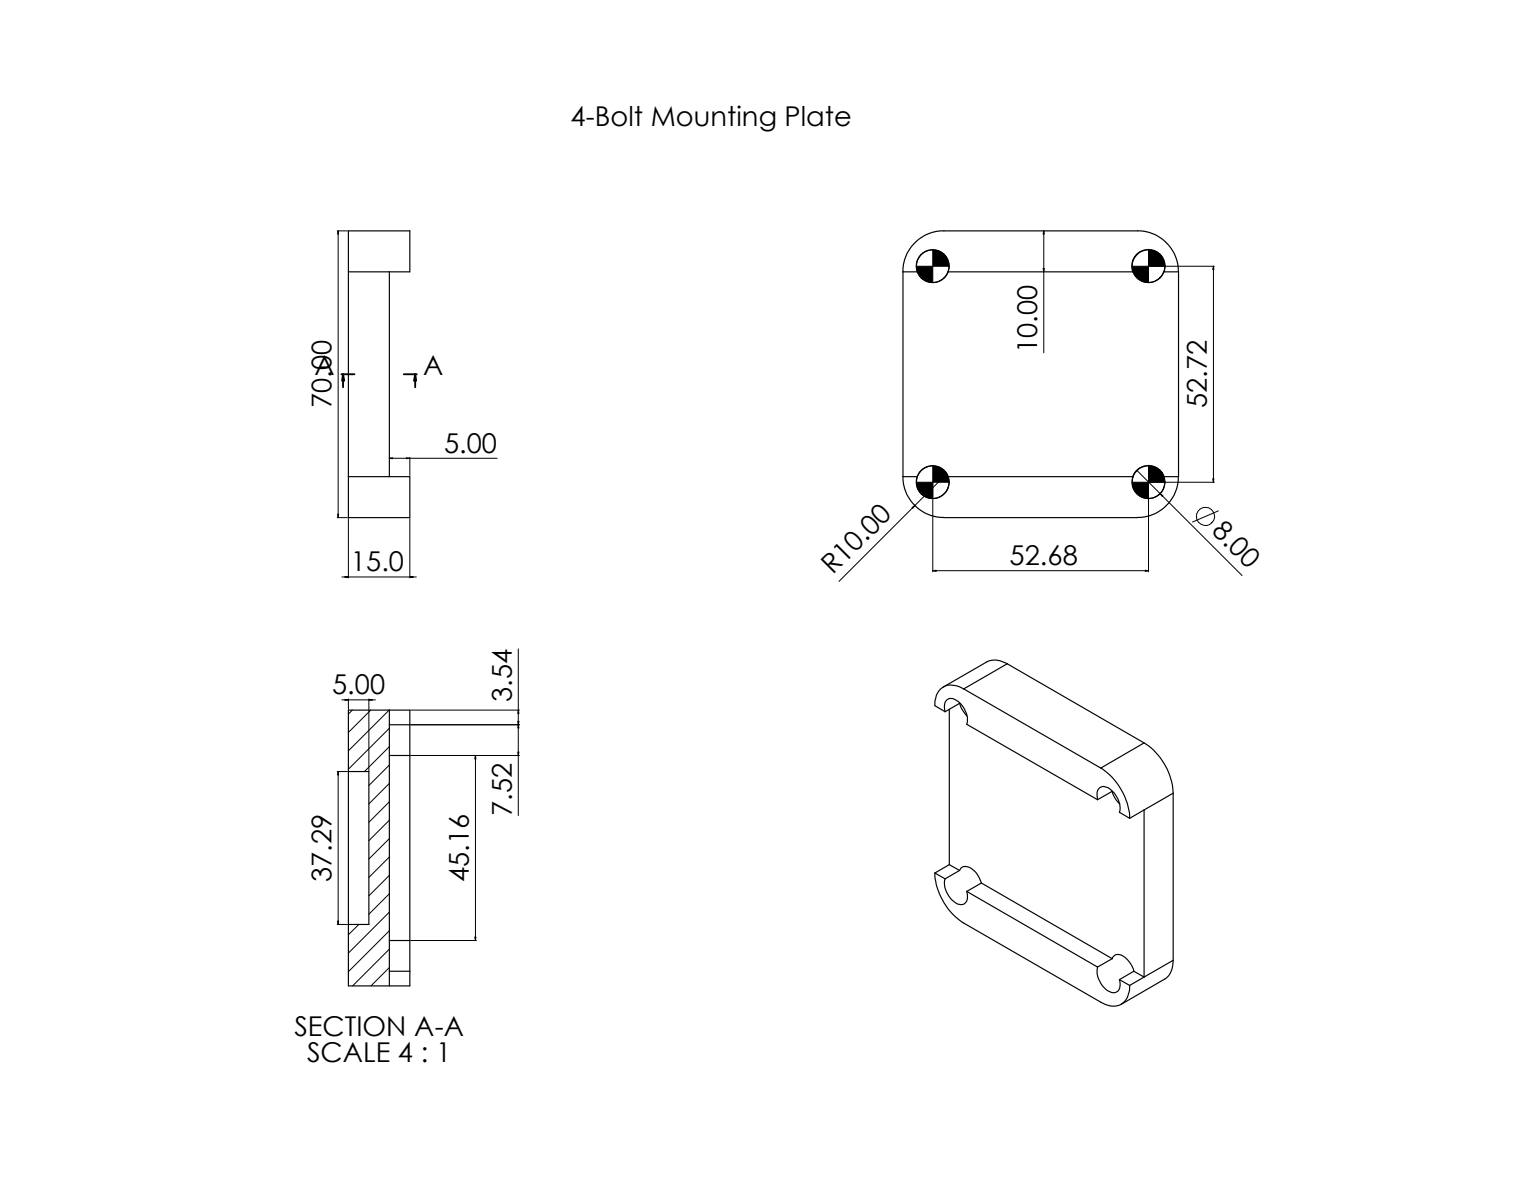
ISO-10303-21;
HEADER;
FILE_DESCRIPTION (('STEP AP214'),
    '1' );
FILE_NAME ('4-Bolt Mounting Plate.step',
    '2026-10-21T18:33:49',
    ( '' ),
    ( '' ),
    'SwSTEP 2.0',
    'SolidWorks 2025',
    '' );
FILE_SCHEMA (( 'AUTOMOTIVE_DESIGN' ));
ENDSEC;

DATA;
#26=AXIS2_PLACEMENT_3D ( 'NONE', #11599, #96, #9826 ) ;
#47=EDGE_CURVE ( 'NONE', #3245, #18159, #14547, .T. ) ;
#49=ORIENTED_EDGE ( 'NONE', *, *, #17445, .T. ) ;
#66=AXIS2_PLACEMENT_3D ( 'NONE', #17711, #16306, #507 ) ;
#94=DIRECTION ( 'NONE',  ( 1.000000000000000000, 0.000000000000000000, -0.000000000000000000 ) ) ;
#96=DIRECTION ( 'NONE',  ( -1.000000000000000000, -0.000000000000000000, -0.000000000000000000 ) ) ;
#118=DIRECTION ( 'NONE',  ( 0.000000000000000000, -0.000000000000000000, 1.000000000000000000 ) ) ;
#119=ORIENTED_EDGE ( 'NONE', *, *, #16367, .F. ) ;
#122=ORIENTED_EDGE ( 'NONE', *, *, #17197, .T. ) ;
#143=CIRCLE ( 'NONE', #12708, 3.999999999999996447 ) ;
#156=EDGE_CURVE ( 'NONE', #14603, #10461, #7800, .T. ) ;
#159=EDGE_CURVE ( 'NONE', #3245, #14275, #15961, .T. ) ;
#162=VERTEX_POINT ( 'NONE', #5272 ) ;
#180=CIRCLE ( 'NONE', #10627, 4.025000000000000355 ) ;
#193=EDGE_LOOP ( 'NONE', ( #119, #17076, #7928, #5091 ) ) ;
#206=ORIENTED_EDGE ( 'NONE', *, *, #10760, .F. ) ;
#214=EDGE_LOOP ( 'NONE', ( #597, #4033, #2043, #6029 ) ) ;
#217=CARTESIAN_POINT ( 'NONE',  ( -97.59262256747317110, 0.3328663868096687350, 25.00000000000000000 ) ) ;
#262=CARTESIAN_POINT ( 'NONE',  ( -92.59262256747321373, 107.8748711238780373, 25.00000000000000000 ) ) ;
#322=AXIS2_PLACEMENT_3D ( 'NONE', #3585, #3405, #3694 ) ;
#334=CARTESIAN_POINT ( 'NONE',  ( -107.5926225674731853, 110.5691553257988460, 22.33417033480641223 ) ) ;
#386=VECTOR ( 'NONE', #13903, 1000.000000000000000 ) ;
#401=VERTEX_POINT ( 'NONE', #7407 ) ;
#404=LINE ( 'NONE', #6368, #15281 ) ;
#488=ORIENTED_EDGE ( 'NONE', *, *, #10760, .T. ) ;
#507=DIRECTION ( 'NONE',  ( 0.000000000000000000, 0.000000000000000000, 1.000000000000000000 ) ) ;
#525=CYLINDRICAL_SURFACE ( 'NONE', #10315, 9.999999999999994671 ) ;
#540=CARTESIAN_POINT ( 'NONE',  ( -107.5926225674731711, 57.88796029049330372, -26.35917033480641436 ) ) ;
#542=ORIENTED_EDGE ( 'NONE', *, *, #17582, .T. ) ;
#545=ORIENTED_EDGE ( 'NONE', *, *, #18144, .T. ) ;
#597=ORIENTED_EDGE ( 'NONE', *, *, #9244, .F. ) ;
#607=FACE_OUTER_BOUND ( 'NONE', #6469, .T. ) ;
#621=ORIENTED_EDGE ( 'NONE', *, *, #9768, .T. ) ;
#623=DIRECTION ( 'NONE',  ( 1.000000000000000000, 2.062304371594500740E-16, 0.000000000000000000 ) ) ;
#665=UNCERTAINTY_MEASURE_WITH_UNIT (LENGTH_MEASURE( 1.000000000000000082E-05 ), #5405, 'distance_accuracy_value', 'NONE');
#676=DIRECTION ( 'NONE',  ( -2.062304371594500740E-16, 1.000000000000000000, 0.000000000000000000 ) ) ;
#682=CYLINDRICAL_SURFACE ( 'NONE', #6960, 3.999999999999996447 ) ;
#700=EDGE_CURVE ( 'NONE', #5246, #2130, #14481, .T. ) ;
#706=VECTOR ( 'NONE', #17635, 1000.000000000000000 ) ;
#734=DIRECTION ( 'NONE',  ( -1.000000000000000000, -0.000000000000000000, -0.000000000000000000 ) ) ;
#735=ORIENTED_EDGE ( 'NONE', *, *, #7900, .T. ) ;
#755=CARTESIAN_POINT ( 'NONE',  ( -107.5926225674731711, 57.88796029049330372, 26.35917033480641436 ) ) ;
#767=EDGE_LOOP ( 'NONE', ( #9960, #18341, #6910, #3598, #2917, #14530, #2645, #13701 ) ) ;
#778=DIRECTION ( 'NONE',  ( 0.000000000000000000, 0.000000000000000000, 1.000000000000000000 ) ) ;
#780=DIRECTION ( 'NONE',  ( -1.000000000000000000, -0.000000000000000000, -0.000000000000000000 ) ) ;
#784=DIRECTION ( 'NONE',  ( -1.000000000000000000, 0.000000000000000000, -0.000000000000000000 ) ) ;
#818=DIRECTION ( 'NONE',  ( 1.000000000000000000, 2.062304371594500494E-16, 0.000000000000000000 ) ) ;
#827=VERTEX_POINT ( 'NONE', #1769 ) ;
#829=DIRECTION ( 'NONE',  ( 0.000000000000000000, 0.000000000000000000, 1.000000000000000000 ) ) ;
#857=VERTEX_POINT ( 'NONE', #3093 ) ;
#873=DIRECTION ( 'NONE',  ( 1.000000000000000000, 2.062304371594500494E-16, 0.000000000000000000 ) ) ;
#877=DIRECTION ( 'NONE',  ( 1.000000000000000000, 2.062304371594500494E-16, -2.775557561562890858E-16 ) ) ;
#878=ORIENTED_EDGE ( 'NONE', *, *, #12466, .F. ) ;
#899=CARTESIAN_POINT ( 'NONE',  ( -92.59262256747318531, 0.3328663868096687350, 25.00000000000000000 ) ) ;
#904=FACE_BOUND ( 'NONE', #13164, .T. ) ;
#909=CARTESIAN_POINT ( 'NONE',  ( -107.5926225674731853, 114.3311569208253786, -25.00000000000000000 ) ) ;
#919=( NAMED_UNIT ( * ) PLANE_ANGLE_UNIT ( ) SI_UNIT ( $, .RADIAN. ) );
#949=VECTOR ( 'NONE', #12099, 1000.000000000000000 ) ;
#961=VERTEX_POINT ( 'NONE', #2238 ) ;
#971=ORIENTED_EDGE ( 'NONE', *, *, #11111, .T. ) ;
#975=AXIS2_PLACEMENT_3D ( 'NONE', #12188, #9288, #4882 ) ;
#980=CARTESIAN_POINT ( 'NONE',  ( -97.59262256747319952, 110.5691553257988460, 26.35917033480641436 ) ) ;
#990=ORIENTED_EDGE ( 'NONE', *, *, #15850, .T. ) ;
#993=EDGE_CURVE ( 'NONE', #9785, #3688, #10294, .T. ) ;
#1005=VECTOR ( 'NONE', #11411, 1000.000000000000114 ) ;
#1009=CARTESIAN_POINT ( 'NONE',  ( -92.59262256747321373, 117.8748711238780515, 25.00000000000000000 ) ) ;
#1012=CARTESIAN_POINT ( 'NONE',  ( -107.5926225674732137, 107.8748711238780373, 35.00000000000000000 ) ) ;
#1020=CIRCLE ( 'NONE', #6697, 9.999999999999994671 ) ;
#1053=EDGE_CURVE ( 'NONE', #17316, #9785, #16350, .T. ) ;
#1062=CARTESIAN_POINT ( 'NONE',  ( -107.5926225674731711, 57.88796029049330372, 26.35917033480641436 ) ) ;
#1075=VECTOR ( 'NONE', #6731, 1000.000000000000114 ) ;
#1078=ORIENTED_EDGE ( 'NONE', *, *, #12131, .F. ) ;
#1081=EDGE_CURVE ( 'NONE', #3688, #13603, #10947, .T. ) ;
#1099=DIRECTION ( 'NONE',  ( 0.000000000000000000, 1.000000000000000000, 0.000000000000000000 ) ) ;
#1119=VERTEX_POINT ( 'NONE', #15330 ) ;
#1122=LINE ( 'NONE', #8417, #18391 ) ;
#1138=EDGE_CURVE ( 'NONE', #162, #13480, #1122, .T. ) ;
#1140=EDGE_CURVE ( 'NONE', #9962, #16099, #6915, .T. ) ;
#1142=DIRECTION ( 'NONE',  ( -2.062304371594500494E-16, 1.000000000000000000, -0.000000000000000000 ) ) ;
#1156=EDGE_LOOP ( 'NONE', ( #16086, #9240, #2898, #2982 ) ) ;
#1160=EDGE_CURVE ( 'NONE', #14280, #401, #8316, .T. ) ;
#1179=CARTESIAN_POINT ( 'NONE',  ( -102.5926225674731853, 102.8748711238780373, -20.00000000000000355 ) ) ;
#1239=DIRECTION ( 'NONE',  ( -1.000000000000000000, -0.000000000000000000, -0.000000000000000000 ) ) ;
#1276=CIRCLE ( 'NONE', #7821, 3.999999999999989786 ) ;
#1314=VECTOR ( 'NONE', #1694, 1000.000000000000000 ) ;
#1334=ORIENTED_EDGE ( 'NONE', *, *, #13295, .F. ) ;
#1336=ORIENTED_EDGE ( 'NONE', *, *, #11789, .F. ) ;
#1342=ADVANCED_FACE ( 'NONE', ( #13350 ), #525, .T. ) ;
#1372=ORIENTED_EDGE ( 'NONE', *, *, #12466, .T. ) ;
#1401=EDGE_CURVE ( 'NONE', #2087, #827, #2426, .T. ) ;
#1433=CARTESIAN_POINT ( 'NONE',  ( -102.5926225674731569, 65.58224449241410525, 20.00000000000000355 ) ) ;
#1436=ORIENTED_EDGE ( 'NONE', *, *, #18437, .F. ) ;
#1446=LINE ( 'NONE', #12590, #11532 ) ;
#1457=CARTESIAN_POINT ( 'NONE',  ( -107.5926225674731853, 110.5691553257988460, 26.35917033480641436 ) ) ;
#1485=( NAMED_UNIT ( * ) PLANE_ANGLE_UNIT ( ) SI_UNIT ( $, .RADIAN. ) );
#1504=ORIENTED_EDGE ( 'NONE', *, *, #7764, .F. ) ;
#1536=AXIS2_PLACEMENT_3D ( 'NONE', #16378, #3567, #17511 ) ;
#1549=CIRCLE ( 'NONE', #5112, 4.000000000000003553 ) ;
#1561=PLANE ( 'NONE',  #12933 ) ;
#1564=VECTOR ( 'NONE', #9130, 1000.000000000000000 ) ;
#1570=AXIS2_PLACEMENT_3D ( 'NONE', #5555, #6963, #6776 ) ;
#1573=VECTOR ( 'NONE', #11269, 1000.000000000000000 ) ;
#1575=CARTESIAN_POINT ( 'NONE',  ( -107.5926225674732137, 117.8748711238780373, 25.00000000000000000 ) ) ;
#1593=CIRCLE ( 'NONE', #3977, 9.999999999999994671 ) ;
#1603=VECTOR ( 'NONE', #6733, 1000.000000000000000 ) ;
#1631=DIRECTION ( 'NONE',  ( -1.000000000000000000, -0.000000000000000000, -0.000000000000000000 ) ) ;
#1632=DIRECTION ( 'NONE',  ( 0.000000000000000000, 1.000000000000000000, 0.000000000000000000 ) ) ;
#1655=DIRECTION ( 'NONE',  ( 1.000000000000000000, 2.062304371594500247E-16, 0.000000000000000000 ) ) ;
#1657=VECTOR ( 'NONE', #15980, 1000.000000000000000 ) ;
#1665=CIRCLE ( 'NONE', #7895, 3.999999999999996447 ) ;
#1694=DIRECTION ( 'NONE',  ( -1.000000000000000000, -2.062304371594500740E-16, -0.000000000000000000 ) ) ;
#1715=PLANE ( 'NONE',  #2686 ) ;
#1717=EDGE_CURVE ( 'NONE', #401, #16431, #11237, .T. ) ;
#1763=DIRECTION ( 'NONE',  ( 1.000000000000000000, 2.062304371594500494E-16, 0.000000000000000000 ) ) ;
#1765=ORIENTED_EDGE ( 'NONE', *, *, #15575, .T. ) ;
#1769=CARTESIAN_POINT ( 'NONE',  ( -107.5676225674731938, 110.5691553257988460, -30.35917033480641791 ) ) ;
#1779=CARTESIAN_POINT ( 'NONE',  ( -97.59262256747318531, 0.3328663868096687350, -25.00000000000000000 ) ) ;
#1789=AXIS2_PLACEMENT_3D ( 'NONE', #17035, #4136, #5539 ) ;
#1809=AXIS2_PLACEMENT_3D ( 'NONE', #16405, #17904, #7814 ) ;
#1811=ORIENTED_EDGE ( 'NONE', *, *, #16462, .T. ) ;
#1847=ORIENTED_EDGE ( 'NONE', *, *, #4139, .T. ) ;
#1866=AXIS2_PLACEMENT_3D ( 'NONE', #9872, #6873, #18396 ) ;
#1910=ORIENTED_EDGE ( 'NONE', *, *, #10499, .F. ) ;
#1920=EDGE_CURVE ( 'NONE', #12847, #10167, #11827, .T. ) ;
#1921=CARTESIAN_POINT ( 'NONE',  ( -107.5926225674731853, 106.8071537307723133, -25.00000000000000000 ) ) ;
#1923=DIRECTION ( 'NONE',  ( -0.000000000000000000, 0.000000000000000000, -1.000000000000000000 ) ) ;
#1926=AXIS2_PLACEMENT_3D ( 'NONE', #18097, #873, #16490 ) ;
#1938=DIRECTION ( 'NONE',  ( -0.000000000000000000, 0.000000000000000000, -1.000000000000000000 ) ) ;
#1944=FACE_BOUND ( 'NONE', #9965, .T. ) ;
#1956=CARTESIAN_POINT ( 'NONE',  ( -92.59262256747318531, -1.909541702982995504E-14, 0.000000000000000000 ) ) ;
#1977=ORIENTED_EDGE ( 'NONE', *, *, #5844, .F. ) ;
#1988=ORIENTED_EDGE ( 'NONE', *, *, #11789, .T. ) ;
#1990=CARTESIAN_POINT ( 'NONE',  ( -107.5926225674731711, 65.58224449241410525, -20.00000000000000355 ) ) ;
#1996=CYLINDRICAL_SURFACE ( 'NONE', #10404, 3.999999999999989786 ) ;
#1997=ORIENTED_EDGE ( 'NONE', *, *, #18461, .F. ) ;
#2003=CARTESIAN_POINT ( 'NONE',  ( -107.5926225674731853, 110.5691553257988460, -26.35917033480641436 ) ) ;
#2004=CARTESIAN_POINT ( 'NONE',  ( -107.5926225674731711, 57.88796029049330372, -26.35917033480641436 ) ) ;
#2017=FACE_OUTER_BOUND ( 'NONE', #11619, .T. ) ;
#2028=DIRECTION ( 'NONE',  ( -0.7071067811865474617, 0.000000000000000000, 0.7071067811865474617 ) ) ;
#2030=AXIS2_PLACEMENT_3D ( 'NONE', #4978, #3296, #784 ) ;
#2032=EDGE_LOOP ( 'NONE', ( #5746, #13506, #14740, #11251, #18492, #14246 ) ) ;
#2043=ORIENTED_EDGE ( 'NONE', *, *, #13295, .T. ) ;
#2045=DIRECTION ( 'NONE',  ( 1.000000000000000000, 2.062304371594500494E-16, -2.775557561562890858E-16 ) ) ;
#2053=EDGE_CURVE ( 'NONE', #3000, #12847, #1593, .T. ) ;
#2069=DIRECTION ( 'NONE',  ( 1.000000000000000000, 2.062304371594500740E-16, 0.000000000000000000 ) ) ;
#2071=FACE_OUTER_BOUND ( 'NONE', #8201, .T. ) ;
#2084=EDGE_CURVE ( 'NONE', #14275, #961, #7845, .T. ) ;
#2087=VERTEX_POINT ( 'NONE', #2415 ) ;
#2121=CARTESIAN_POINT ( 'NONE',  ( -107.5926225674731711, -2.218887358722170814E-14, 0.000000000000000000 ) ) ;
#2127=VECTOR ( 'NONE', #17715, 1000.000000000000000 ) ;
#2130=VERTEX_POINT ( 'NONE', #9249 ) ;
#2134=ORIENTED_EDGE ( 'NONE', *, *, #4548, .F. ) ;
#2149=VECTOR ( 'NONE', #4447, 1000.000000000000000 ) ;
#2150=DIRECTION ( 'NONE',  ( -1.000000000000000000, -2.062304371594500494E-16, -0.000000000000000000 ) ) ;
#2184=EDGE_CURVE ( 'NONE', #18220, #11731, #18040, .T. ) ;
#2196=ORIENTED_EDGE ( 'NONE', *, *, #12976, .T. ) ;
#2210=DIRECTION ( 'NONE',  ( 0.000000000000000000, 1.000000000000000000, 0.000000000000000000 ) ) ;
#2216=PLANE ( 'NONE',  #2717 ) ;
#2221=CIRCLE ( 'NONE', #8525, 9.999999999999994671 ) ;
#2224=DIRECTION ( 'NONE',  ( 0.000000000000000000, 0.000000000000000000, 1.000000000000000000 ) ) ;
#2238=CARTESIAN_POINT ( 'NONE',  ( -92.59262256747319952, 54.12595869546677818, 25.00000000000000000 ) ) ;
#2247=VERTEX_POINT ( 'NONE', #6623 ) ;
#2257=DIRECTION ( 'NONE',  ( 0.000000000000000000, 0.000000000000000000, 1.000000000000000000 ) ) ;
#2258=FACE_OUTER_BOUND ( 'NONE', #4938, .T. ) ;
#2260=CARTESIAN_POINT ( 'NONE',  ( -92.59262256747321373, 114.3311569208253786, 25.00000000000000000 ) ) ;
#2277=CARTESIAN_POINT ( 'NONE',  ( -92.59262256747319952, 60.58224449241411946, -35.00000000000000000 ) ) ;
#2287=DIRECTION ( 'NONE',  ( -0.000000000000000000, -0.000000000000000000, 1.000000000000000000 ) ) ;
#2291=EDGE_CURVE ( 'NONE', #9785, #11807, #12812, .T. ) ;
#2293=EDGE_CURVE ( 'NONE', #15245, #16207, #12739, .T. ) ;
#2310=CARTESIAN_POINT ( 'NONE',  ( -97.59262256747318531, 50.58224449241411236, 25.00000000000000000 ) ) ;
#2325=CARTESIAN_POINT ( 'NONE',  ( -92.59262256747321373, 107.8748711238780373, -25.00000000000000000 ) ) ;
#2335=ORIENTED_EDGE ( 'NONE', *, *, #1160, .T. ) ;
#2337=UNCERTAINTY_MEASURE_WITH_UNIT (LENGTH_MEASURE( 1.000000000000000082E-05 ), #8875, 'distance_accuracy_value', 'NONE');
#2342=CARTESIAN_POINT ( 'NONE',  ( -92.59262256747318531, 0.3328663868096687350, -25.00000000000000000 ) ) ;
#2348=DIRECTION ( 'NONE',  ( 0.000000000000000000, 1.000000000000000000, 0.000000000000000000 ) ) ;
#2351=DIRECTION ( 'NONE',  ( 0.000000000000000000, 0.000000000000000000, 1.000000000000000000 ) ) ;
#2363=PRODUCT_CONTEXT ( 'NONE', #7518, 'mechanical' ) ;
#2375=EDGE_CURVE ( 'NONE', #15333, #12447, #11163, .T. ) ;
#2415=CARTESIAN_POINT ( 'NONE',  ( -92.59262256747321373, 110.5691553257988460, -30.35917033480641081 ) ) ;
#2426=LINE ( 'NONE', #13660, #11813 ) ;
#2456=AXIS2_PLACEMENT_3D ( 'NONE', #15865, #7367, #13080 ) ;
#2480=LINE ( 'NONE', #13906, #3660 ) ;
#2498=CARTESIAN_POINT ( 'NONE',  ( -107.5926225674731711, 57.88796029049330372, 30.38417033480641294 ) ) ;
#2518=EDGE_CURVE ( 'NONE', #10461, #15190, #6209, .T. ) ;
#2519=DIRECTION ( 'NONE',  ( -2.062304371594500494E-16, 1.000000000000000000, -0.000000000000000000 ) ) ;
#2526=VECTOR ( 'NONE', #7508, 1000.000000000000000 ) ;
#2543=ORIENTED_EDGE ( 'NONE', *, *, #12676, .T. ) ;
#2545=ORIENTED_EDGE ( 'NONE', *, *, #2518, .T. ) ;
#2553=DIRECTION ( 'NONE',  ( 0.000000000000000000, 0.000000000000000000, 1.000000000000000000 ) ) ;
#2562=CARTESIAN_POINT ( 'NONE',  ( -107.5926225674732137, 107.8748711238780373, 25.00000000000000000 ) ) ;
#2636=DIRECTION ( 'NONE',  ( 0.000000000000000000, 0.000000000000000000, 1.000000000000000000 ) ) ;
#2645=ORIENTED_EDGE ( 'NONE', *, *, #12131, .T. ) ;
#2647=LINE ( 'NONE', #9766, #8665 ) ;
#2672=DIRECTION ( 'NONE',  ( -1.000000000000000000, -2.062304371594500247E-16, -0.000000000000000000 ) ) ;
#2686=AXIS2_PLACEMENT_3D ( 'NONE', #12788, #5747, #12874 ) ;
#2690=CIRCLE ( 'NONE', #11362, 3.999999999999996447 ) ;
#2717=AXIS2_PLACEMENT_3D ( 'NONE', #2121, #818, #7930 ) ;
#2730=DIRECTION ( 'NONE',  ( 0.000000000000000000, 1.000000000000000000, 0.000000000000000000 ) ) ;
#2736=CARTESIAN_POINT ( 'NONE',  ( -97.59262256747318531, 61.64996188551983636, 25.00000000000000000 ) ) ;
#2762=DIRECTION ( 'NONE',  ( 1.000000000000000000, 0.000000000000000000, 0.000000000000000000 ) ) ;
#2797=VERTEX_POINT ( 'NONE', #10792 ) ;
#2805=VECTOR ( 'NONE', #1142, 1000.000000000000000 ) ;
#2818=EDGE_LOOP ( 'NONE', ( #6948, #15133, #122, #13825, #10648, #488 ) ) ;
#2823=ORIENTED_EDGE ( 'NONE', *, *, #10499, .T. ) ;
#2859=CARTESIAN_POINT ( 'NONE',  ( -107.5926225674731995, 60.58224449241411946, 35.00000000000000000 ) ) ;
#2866=DIRECTION ( 'NONE',  ( 2.062304371594500740E-16, -1.000000000000000000, 0.000000000000000000 ) ) ;
#2867=VERTEX_POINT ( 'NONE', #5554 ) ;
#2883=CARTESIAN_POINT ( 'NONE',  ( -102.5926225674731853, 102.8748711238780373, -20.00000000000000355 ) ) ;
#2898=ORIENTED_EDGE ( 'NONE', *, *, #3063, .T. ) ;
#2914=ORIENTED_EDGE ( 'NONE', *, *, #12976, .F. ) ;
#2917=ORIENTED_EDGE ( 'NONE', *, *, #17381, .T. ) ;
#2926=ORIENTED_EDGE ( 'NONE', *, *, #15850, .F. ) ;
#2955=DIRECTION ( 'NONE',  ( 0.000000000000000000, 0.000000000000000000, 1.000000000000000000 ) ) ;
#2968=DIRECTION ( 'NONE',  ( 1.000000000000000000, 2.062304371594500740E-16, 0.000000000000000000 ) ) ;
#2982=ORIENTED_EDGE ( 'NONE', *, *, #6512, .F. ) ;
#2989=ORIENTED_EDGE ( 'NONE', *, *, #14091, .T. ) ;
#3000=VERTEX_POINT ( 'NONE', #15752 ) ;
#3006=AXIS2_PLACEMENT_3D ( 'NONE', #7206, #12924, #15632 ) ;
#3009=CARTESIAN_POINT ( 'NONE',  ( -107.5926225674731853, 60.58224449241411946, -25.00000000000000000 ) ) ;
#3038=VERTEX_POINT ( 'NONE', #7333 ) ;
#3051=CIRCLE ( 'NONE', #66, 3.999999999999996447 ) ;
#3054=LINE ( 'NONE', #8946, #2149 ) ;
#3063=EDGE_CURVE ( 'NONE', #5132, #10265, #10131, .T. ) ;
#3082=VECTOR ( 'NONE', #15623, 1000.000000000000000 ) ;
#3086=VERTEX_POINT ( 'NONE', #14607 ) ;
#3092=ORIENTED_EDGE ( 'NONE', *, *, #18301, .T. ) ;
#3093=CARTESIAN_POINT ( 'NONE',  ( -97.59262256747319952, 57.88796029049330372, -22.35917033480642502 ) ) ;
#3094=LINE ( 'NONE', #13197, #3680 ) ;
#3108=ORIENTED_EDGE ( 'NONE', *, *, #16825, .T. ) ;
#3114=ADVANCED_FACE ( 'NONE', ( #2071 ), #17585, .F. ) ;
#3142=VECTOR ( 'NONE', #12538, 1000.000000000000000 ) ;
#3154=ORIENTED_EDGE ( 'NONE', *, *, #11457, .T. ) ;
#3158=LINE ( 'NONE', #5771, #7043 ) ;
#3168=DIRECTION ( 'NONE',  ( -1.000000000000000000, -2.062304371594500247E-16, -0.000000000000000000 ) ) ;
#3212=CARTESIAN_POINT ( 'NONE',  ( -92.59262256747319952, 57.88796029049330372, -26.35917033480641436 ) ) ;
#3224=DIRECTION ( 'NONE',  ( 2.775557561562891351E-16, 0.000000000000000000, 1.000000000000000000 ) ) ;
#3245=VERTEX_POINT ( 'NONE', #14052 ) ;
#3258=ADVANCED_FACE ( 'NONE', ( #2258 ), #3709, .F. ) ;
#3262=LINE ( 'NONE', #11872, #15926 ) ;
#3296=DIRECTION ( 'NONE',  ( 0.000000000000000000, 0.000000000000000000, -1.000000000000000000 ) ) ;
#3301=CIRCLE ( 'NONE', #3609, 9.999999999999994671 ) ;
#3327=DIRECTION ( 'NONE',  ( 1.000000000000000000, 2.062304371594500494E-16, 0.000000000000000000 ) ) ;
#3355=AXIS2_PLACEMENT_3D ( 'NONE', #2342, #1938, #7645 ) ;
#3356=CYLINDRICAL_SURFACE ( 'NONE', #14932, 9.999999999999994671 ) ;
#3360=FACE_OUTER_BOUND ( 'NONE', #10097, .T. ) ;
#3378=ORIENTED_EDGE ( 'NONE', *, *, #6649, .F. ) ;
#3397=EDGE_LOOP ( 'NONE', ( #5138, #18295, #8550, #1436 ) ) ;
#3400=AXIS2_PLACEMENT_3D ( 'NONE', #2004, #17440, #4801 ) ;
#3405=DIRECTION ( 'NONE',  ( -1.000000000000000000, -0.000000000000000000, -0.000000000000000000 ) ) ;
#3429=DIRECTION ( 'NONE',  ( 0.000000000000000000, 1.000000000000000000, 0.000000000000000000 ) ) ;
#3435=LINE ( 'NONE', #7557, #3451 ) ;
#3447=CARTESIAN_POINT ( 'NONE',  ( -92.59262256747318531, 50.58224449241411236, 25.00000000000000000 ) ) ;
#3451=VECTOR ( 'NONE', #2028, 1000.000000000000114 ) ;
#3458=DIRECTION ( 'NONE',  ( 0.000000000000000000, 1.734723475976811433E-15, 1.000000000000000000 ) ) ;
#3467=DIRECTION ( 'NONE',  ( -7.442644330182800165E-16, 1.000000000000000000, 0.000000000000000000 ) ) ;
#3498=CARTESIAN_POINT ( 'NONE',  ( -107.5926225674731853, 102.8748711238780373, 20.00000000000000355 ) ) ;
#3500=CARTESIAN_POINT ( 'NONE',  ( -107.5926225674732137, 117.8748711238780373, 35.00000000000000000 ) ) ;
#3504=EDGE_LOOP ( 'NONE', ( #9305, #206, #17313, #14357 ) ) ;
#3506=FACE_OUTER_BOUND ( 'NONE', #7755, .T. ) ;
#3527=EDGE_CURVE ( 'NONE', #857, #3086, #11874, .T. ) ;
#3567=DIRECTION ( 'NONE',  ( -1.000000000000000000, -0.000000000000000000, -0.000000000000000000 ) ) ;
#3568=LINE ( 'NONE', #1990, #6002 ) ;
#3576=AXIS2_PLACEMENT_3D ( 'NONE', #1433, #118, #11615 ) ;
#3584=EDGE_LOOP ( 'NONE', ( #11012, #6454, #17245, #11816 ) ) ;
#3585=CARTESIAN_POINT ( 'NONE',  ( -107.5676225674731654, 57.88796029049330372, 26.35917033480641436 ) ) ;
#3589=CARTESIAN_POINT ( 'NONE',  ( -92.59262256747318531, 0.3328663868096687350, -25.00000000000000000 ) ) ;
#3598=ORIENTED_EDGE ( 'NONE', *, *, #17958, .T. ) ;
#3603=CARTESIAN_POINT ( 'NONE',  ( -107.5926225674731995, 60.58224449241411946, 25.00000000000000000 ) ) ;
#3609=AXIS2_PLACEMENT_3D ( 'NONE', #4256, #4346, #17241 ) ;
#3621=CARTESIAN_POINT ( 'NONE',  ( -107.5926225674731711, 57.88796029049330372, -22.33417033480641223 ) ) ;
#3632=CARTESIAN_POINT ( 'NONE',  ( -107.5926225674732137, 117.8748711238780373, 25.00000000000000000 ) ) ;
#3640=ORIENTED_EDGE ( 'NONE', *, *, #9768, .F. ) ;
#3660=VECTOR ( 'NONE', #2672, 1000.000000000000000 ) ;
#3680=VECTOR ( 'NONE', #10466, 1000.000000000000000 ) ;
#3688=VERTEX_POINT ( 'NONE', #16117 ) ;
#3693=ORIENTED_EDGE ( 'NONE', *, *, #2291, .T. ) ;
#3694=DIRECTION ( 'NONE',  ( 0.000000000000000000, 0.000000000000000000, 1.000000000000000000 ) ) ;
#3695=( GEOMETRIC_REPRESENTATION_CONTEXT ( 3 ) GLOBAL_UNCERTAINTY_ASSIGNED_CONTEXT ( ( #2337 ) ) GLOBAL_UNIT_ASSIGNED_CONTEXT ( ( #8875, #1485, #17279 ) ) REPRESENTATION_CONTEXT ( 'NONE', 'WORKASPACE' ) );
#3706=EDGE_LOOP ( 'NONE', ( #10881, #13062, #5823, #9646, #13348, #17339 ) ) ;
#3709=CONICAL_SURFACE ( 'NONE', #16848, 4.025000000000000355, 0.7853981633975870569 ) ;
#3718=FACE_BOUND ( 'NONE', #9187, .T. ) ;
#3727=CARTESIAN_POINT ( 'NONE',  ( -107.5926225674731853, 110.5691553257988460, -30.38417033480641294 ) ) ;
#3732=EDGE_CURVE ( 'NONE', #1119, #13480, #5856, .T. ) ;
#3737=AXIS2_PLACEMENT_3D ( 'NONE', #2325, #8031, #18349 ) ;
#3756=CARTESIAN_POINT ( 'NONE',  ( -92.59262256747319952, 50.58224449241411236, -25.00000000000000000 ) ) ;
#3758=DIRECTION ( 'NONE',  ( -1.000000000000000000, -0.000000000000000000, -0.000000000000000000 ) ) ;
#3807=ORIENTED_EDGE ( 'NONE', *, *, #17495, .T. ) ;
#3821=VERTEX_POINT ( 'NONE', #8663 ) ;
#3823=CYLINDRICAL_SURFACE ( 'NONE', #8769, 3.999999999999996447 ) ;
#3828=PLANE ( 'NONE',  #5534 ) ;
#3845=DIRECTION ( 'NONE',  ( 0.000000000000000000, 0.000000000000000000, 1.000000000000000000 ) ) ;
#3874=AXIS2_PLACEMENT_3D ( 'NONE', #1179, #4081, #14088 ) ;
#3881=EDGE_LOOP ( 'NONE', ( #3378, #11988, #4276, #11600, #8921 ) ) ;
#3887=EDGE_LOOP ( 'NONE', ( #16536, #6308, #10227, #10193 ) ) ;
#3906=CIRCLE ( 'NONE', #26, 4.025000000000000355 ) ;
#3908=ADVANCED_FACE ( 'NONE', ( #16885 ), #16779, .F. ) ;
#3937=CARTESIAN_POINT ( 'NONE',  ( -107.5926225674731711, 57.88796029049330372, -26.35917033480641436 ) ) ;
#3977=AXIS2_PLACEMENT_3D ( 'NONE', #9379, #7880, #2348 ) ;
#3994=ORIENTED_EDGE ( 'NONE', *, *, #12676, .F. ) ;
#4019=LINE ( 'NONE', #13939, #13536 ) ;
#4022=CONICAL_SURFACE ( 'NONE', #14477, 4.025000000000000355, 0.7853981633974482790 ) ;
#4023=ADVANCED_FACE ( 'NONE', ( #17330 ), #1715, .T. ) ;
#4033=ORIENTED_EDGE ( 'NONE', *, *, #4271, .T. ) ;
#4034=ADVANCED_FACE ( 'NONE', ( #18484 ), #12974, .F. ) ;
#4040=CARTESIAN_POINT ( 'NONE',  ( -107.5926225674731711, 65.58224449241410525, -20.00000000000000355 ) ) ;
#4051=FACE_OUTER_BOUND ( 'NONE', #3584, .T. ) ;
#4081=DIRECTION ( 'NONE',  ( 0.000000000000000000, 0.000000000000000000, -1.000000000000000000 ) ) ;
#4096=ORIENTED_EDGE ( 'NONE', *, *, #8223, .F. ) ;
#4115=ORIENTED_EDGE ( 'NONE', *, *, #1160, .F. ) ;
#4119=LINE ( 'NONE', #18051, #9025 ) ;
#4136=DIRECTION ( 'NONE',  ( -1.000000000000000000, -0.000000000000000000, -0.000000000000000000 ) ) ;
#4139=EDGE_CURVE ( 'NONE', #7061, #16660, #14904, .T. ) ;
#4156=ORIENTED_EDGE ( 'NONE', *, *, #3527, .T. ) ;
#4192=DIRECTION ( 'NONE',  ( -1.000000000000000000, -2.062304371594500740E-16, -0.000000000000000000 ) ) ;
#4202=CARTESIAN_POINT ( 'NONE',  ( -107.5926225674731711, 57.88796029049330372, 22.33417033480641223 ) ) ;
#4225=CARTESIAN_POINT ( 'NONE',  ( -107.5926225674731853, 110.5691553257988460, 26.35917033480641436 ) ) ;
#4249=VECTOR ( 'NONE', #734, 1000.000000000000000 ) ;
#4256=CARTESIAN_POINT ( 'NONE',  ( -107.5926225674731853, 60.58224449241411946, 25.00000000000000000 ) ) ;
#4259=LINE ( 'NONE', #12871, #386 ) ;
#4271=EDGE_CURVE ( 'NONE', #827, #5082, #2647, .T. ) ;
#4276=ORIENTED_EDGE ( 'NONE', *, *, #10870, .F. ) ;
#4344=LINE ( 'NONE', #16879, #9401 ) ;
#4346=DIRECTION ( 'NONE',  ( -1.000000000000000000, -2.062304371594500494E-16, -0.000000000000000000 ) ) ;
#4386=SHAPE_REPRESENTATION_RELATIONSHIP ( 'NONE' , 'NONE' ,  #16862, #14171 ) ;
#4409=ORIENTED_EDGE ( 'NONE', *, *, #2293, .F. ) ;
#4435=ADVANCED_FACE ( 'NONE', ( #14519 ), #14256, .F. ) ;
#4437=CARTESIAN_POINT ( 'NONE',  ( -102.5926225674731569, 65.58224449241410525, -20.00000000000000355 ) ) ;
#4440=CARTESIAN_POINT ( 'NONE',  ( -97.59262256747321373, 117.8748711238780515, -25.00000000000000000 ) ) ;
#4447=DIRECTION ( 'NONE',  ( 7.442644330182800165E-16, -1.000000000000000000, 0.000000000000000000 ) ) ;
#4526=DIRECTION ( 'NONE',  ( -2.062304371594500494E-16, 1.000000000000000000, -0.000000000000000000 ) ) ;
#4548=EDGE_CURVE ( 'NONE', #14915, #12020, #7761, .T. ) ;
#4550=AXIS2_PLACEMENT_3D ( 'NONE', #9685, #9781, #7074 ) ;
#4620=ORIENTED_EDGE ( 'NONE', *, *, #156, .T. ) ;
#4695=ORIENTED_EDGE ( 'NONE', *, *, #12077, .F. ) ;
#4700=VERTEX_POINT ( 'NONE', #12365 ) ;
#4716=VECTOR ( 'NONE', #8353, 1000.000000000000000 ) ;
#4728=ORIENTED_EDGE ( 'NONE', *, *, #17495, .F. ) ;
#4756=CIRCLE ( 'NONE', #1789, 3.999999999999996447 ) ;
#4771=DIRECTION ( 'NONE',  ( -1.000000000000000000, -2.062304371594500740E-16, 0.000000000000000000 ) ) ;
#4791=ORIENTED_EDGE ( 'NONE', *, *, #18301, .F. ) ;
#4792=VECTOR ( 'NONE', #1631, 1000.000000000000000 ) ;
#4793=CARTESIAN_POINT ( 'NONE',  ( -92.59262256747321373, 117.8748711238780373, 35.00000000000000000 ) ) ;
#4795=EDGE_CURVE ( 'NONE', #2797, #11084, #8389, .T. ) ;
#4801=DIRECTION ( 'NONE',  ( 0.000000000000000000, 0.000000000000000000, 1.000000000000000000 ) ) ;
#4803=EDGE_CURVE ( 'NONE', #11561, #2867, #3906, .T. ) ;
#4805=ORIENTED_EDGE ( 'NONE', *, *, #11565, .T. ) ;
#4809=CARTESIAN_POINT ( 'NONE',  ( -107.5926225674731853, 50.58224449241411236, 35.00000000000000000 ) ) ;
#4819=DIRECTION ( 'NONE',  ( -1.000000000000000000, -0.000000000000000000, -0.000000000000000000 ) ) ;
#4847=CARTESIAN_POINT ( 'NONE',  ( -107.5926225674731853, 110.5691553257988460, 30.35917033480641081 ) ) ;
#4851=LINE ( 'NONE', #15234, #11381 ) ;
#4854=ORIENTED_EDGE ( 'NONE', *, *, #1717, .T. ) ;
#4875=ORIENTED_EDGE ( 'NONE', *, *, #8488, .F. ) ;
#4880=DIRECTION ( 'NONE',  ( -1.000000000000000000, -0.000000000000000000, -0.000000000000000000 ) ) ;
#4882=DIRECTION ( 'NONE',  ( 0.000000000000000000, 1.000000000000000000, 0.000000000000000000 ) ) ;
#4907=CARTESIAN_POINT ( 'NONE',  ( -107.5926225674731711, 54.12595869546677818, -25.00000000000000000 ) ) ;
#4910=LINE ( 'NONE', #4809, #7604 ) ;
#4937=LINE ( 'NONE', #1012, #12629 ) ;
#4938=EDGE_LOOP ( 'NONE', ( #9520, #17217, #16566, #17818 ) ) ;
#4972=CARTESIAN_POINT ( 'NONE',  ( -107.5926225674731853, 110.5691553257988460, -26.35917033480641436 ) ) ;
#4978=CARTESIAN_POINT ( 'NONE',  ( -107.5926225674732137, 117.8748711238780373, 35.00000000000000000 ) ) ;
#4980=PRODUCT_DEFINITION ( 'UNKNOWN', '', #7010, #18457 ) ;
#4997=ORIENTED_EDGE ( 'NONE', *, *, #5154, .T. ) ;
#5044=CARTESIAN_POINT ( 'NONE',  ( -97.59262256747318531, 0.3328663868096687350, -25.00000000000000000 ) ) ;
#5058=PLANE ( 'NONE',  #10810 ) ;
#5061=LINE ( 'NONE', #16379, #949 ) ;
#5066=EDGE_LOOP ( 'NONE', ( #5354, #2926, #7190, #10376 ) ) ;
#5071=ORIENTED_EDGE ( 'NONE', *, *, #15206, .F. ) ;
#5081=AXIS2_PLACEMENT_3D ( 'NONE', #11116, #15500, #11305 ) ;
#5082=VERTEX_POINT ( 'NONE', #3727 ) ;
#5091=ORIENTED_EDGE ( 'NONE', *, *, #17173, .T. ) ;
#5112=AXIS2_PLACEMENT_3D ( 'NONE', #5254, #10969, #8159 ) ;
#5113=DIRECTION ( 'NONE',  ( 0.000000000000000000, 0.000000000000000000, 1.000000000000000000 ) ) ;
#5132=VERTEX_POINT ( 'NONE', #2310 ) ;
#5135=AXIS2_PLACEMENT_3D ( 'NONE', #3589, #1923, #7532 ) ;
#5138=ORIENTED_EDGE ( 'NONE', *, *, #11144, .T. ) ;
#5153=FACE_OUTER_BOUND ( 'NONE', #3397, .T. ) ;
#5154=EDGE_CURVE ( 'NONE', #7063, #401, #14296, .T. ) ;
#5161=FACE_OUTER_BOUND ( 'NONE', #6766, .T. ) ;
#5182=CARTESIAN_POINT ( 'NONE',  ( -107.5926225674731711, 57.88796029049330372, 30.38417033480641294 ) ) ;
#5246=VERTEX_POINT ( 'NONE', #5677 ) ;
#5250=LINE ( 'NONE', #3756, #13820 ) ;
#5254=CARTESIAN_POINT ( 'NONE',  ( -107.5676225674731938, 110.5691553257988460, -26.35917033480641436 ) ) ;
#5272=CARTESIAN_POINT ( 'NONE',  ( -97.59262256747319952, 114.3311569208253786, 25.00000000000000000 ) ) ;
#5287=FACE_OUTER_BOUND ( 'NONE', #1156, .T. ) ;
#5290=FACE_OUTER_BOUND ( 'NONE', #3504, .T. ) ;
#5325=ADVANCED_FACE ( 'NONE', ( #14806 ), #9387, .F. ) ;
#5354=ORIENTED_EDGE ( 'NONE', *, *, #16926, .T. ) ;
#5368=ADVANCED_FACE ( 'NONE', ( #14987 ), #1996, .F. ) ;
#5405=( LENGTH_UNIT ( ) NAMED_UNIT ( * ) SI_UNIT ( .MILLI., .METRE. ) );
#5427=AXIS2_PLACEMENT_3D ( 'NONE', #4972, #4880, #9378 ) ;
#5428=AXIS2_PLACEMENT_3D ( 'NONE', #18263, #5437, #15459 ) ;
#5437=DIRECTION ( 'NONE',  ( -1.000000000000000000, -0.000000000000000000, -0.000000000000000000 ) ) ;
#5445=VECTOR ( 'NONE', #17209, 1000.000000000000000 ) ;
#5448=LINE ( 'NONE', #6770, #4716 ) ;
#5452=AXIS2_PLACEMENT_3D ( 'NONE', #17783, #2257, #6360 ) ;
#5513=CARTESIAN_POINT ( 'NONE',  ( -107.5926225674731853, 110.5691553257988460, -26.35917033480641436 ) ) ;
#5514=EDGE_CURVE ( 'NONE', #12447, #2797, #5448, .T. ) ;
#5534=AXIS2_PLACEMENT_3D ( 'NONE', #9352, #16722, #10951 ) ;
#5539=DIRECTION ( 'NONE',  ( 0.000000000000000000, 0.000000000000000000, 1.000000000000000000 ) ) ;
#5541=ORIENTED_EDGE ( 'NONE', *, *, #17734, .T. ) ;
#5554=CARTESIAN_POINT ( 'NONE',  ( -107.5926225674731711, 57.88796029049330372, 22.33417033480641223 ) ) ;
#5555=CARTESIAN_POINT ( 'NONE',  ( -92.59262256747321373, 110.5691553257988460, 26.35917033480641436 ) ) ;
#5605=LINE ( 'NONE', #12823, #5445 ) ;
#5658=CARTESIAN_POINT ( 'NONE',  ( -92.59262256747319952, 60.58224449241411946, -25.00000000000000000 ) ) ;
#5677=CARTESIAN_POINT ( 'NONE',  ( -107.5926225674731711, 57.88796029049330372, -30.38417033480641294 ) ) ;
#5688=EDGE_LOOP ( 'NONE', ( #1847, #1765, #12868, #11563, #10625, #11328 ) ) ;
#5694=ORIENTED_EDGE ( 'NONE', *, *, #13618, .F. ) ;
#5716=CARTESIAN_POINT ( 'NONE',  ( -92.59262256747319952, 54.12595869546677818, -25.00000000000000000 ) ) ;
#5745=CARTESIAN_POINT ( 'NONE',  ( -97.59262256747321373, 110.5691553257988460, -22.35917033480641791 ) ) ;
#5746=ORIENTED_EDGE ( 'NONE', *, *, #10396, .F. ) ;
#5747=DIRECTION ( 'NONE',  ( -1.000000000000000000, -7.442644330182800165E-16, 0.000000000000000000 ) ) ;
#5752=FACE_OUTER_BOUND ( 'NONE', #17274, .T. ) ;
#5766=CONICAL_SURFACE ( 'NONE', #8157, 4.025000000000000355, 0.7853981633975870569 ) ;
#5771=CARTESIAN_POINT ( 'NONE',  ( -107.5926225674731995, 60.58224449241411946, 35.00000000000000000 ) ) ;
#5777=VECTOR ( 'NONE', #4526, 1000.000000000000000 ) ;
#5781=CARTESIAN_POINT ( 'NONE',  ( 0.000000000000000000, 0.000000000000000000, 0.000000000000000000 ) ) ;
#5810=VECTOR ( 'NONE', #13691, 1000.000000000000000 ) ;
#5815=ORIENTED_EDGE ( 'NONE', *, *, #10396, .T. ) ;
#5819=AXIS2_PLACEMENT_3D ( 'NONE', #12066, #7946, #10465 ) ;
#5823=ORIENTED_EDGE ( 'NONE', *, *, #6637, .T. ) ;
#5844=EDGE_CURVE ( 'NONE', #17429, #7061, #8245, .T. ) ;
#5856=LINE ( 'NONE', #4440, #13717 ) ;
#5923=CARTESIAN_POINT ( 'NONE',  ( -92.59262256747318531, 0.3328663868096687350, -25.00000000000000000 ) ) ;
#5929=ADVANCED_FACE ( 'NONE', ( #15060 ), #13857, .F. ) ;
#5944=ORIENTED_EDGE ( 'NONE', *, *, #156, .F. ) ;
#5978=ORIENTED_EDGE ( 'NONE', *, *, #17822, .F. ) ;
#5982=ORIENTED_EDGE ( 'NONE', *, *, #13255, .F. ) ;
#6002=VECTOR ( 'NONE', #778, 1000.000000000000000 ) ;
#6006=CARTESIAN_POINT ( 'NONE',  ( -97.59262256747317110, 0.3328663868096687350, 25.00000000000000000 ) ) ;
#6013=CARTESIAN_POINT ( 'NONE',  ( -107.5676225674731654, 57.88796029049330372, 22.35917033480641791 ) ) ;
#6018=ORIENTED_EDGE ( 'NONE', *, *, #4803, .T. ) ;
#6027=CARTESIAN_POINT ( 'NONE',  ( -97.59262256747319952, 117.8748711238780373, 25.00000000000000000 ) ) ;
#6029=ORIENTED_EDGE ( 'NONE', *, *, #12602, .F. ) ;
#6035=CIRCLE ( 'NONE', #11148, 4.025000000000000355 ) ;
#6037=DIRECTION ( 'NONE',  ( 0.000000000000000000, 0.000000000000000000, 1.000000000000000000 ) ) ;
#6052=CIRCLE ( 'NONE', #12347, 3.999999999999989786 ) ;
#6123=ORIENTED_EDGE ( 'NONE', *, *, #7992, .T. ) ;
#6148=CARTESIAN_POINT ( 'NONE',  ( -92.59262256747321373, 107.8748711238780373, 35.00000000000000000 ) ) ;
#6158=FACE_OUTER_BOUND ( 'NONE', #15357, .T. ) ;
#6209=LINE ( 'NONE', #6496, #8497 ) ;
#6221=FACE_OUTER_BOUND ( 'NONE', #767, .T. ) ;
#6235=MANIFOLD_SOLID_BREP ( 'Cut-Extrude9', #7289 ) ;
#6240=DIRECTION ( 'NONE',  ( 0.000000000000000000, 1.000000000000000000, 0.000000000000000000 ) ) ;
#6263=CARTESIAN_POINT ( 'NONE',  ( -107.5926225674731853, 110.5691553257988460, -22.33417033480641223 ) ) ;
#6273=EDGE_CURVE ( 'NONE', #5132, #11466, #7183, .T. ) ;
#6301=CONICAL_SURFACE ( 'NONE', #9912, 4.025000000000000355, 0.7853981633975870569 ) ;
#6308=ORIENTED_EDGE ( 'NONE', *, *, #3732, .F. ) ;
#6357=VECTOR ( 'NONE', #2955, 1000.000000000000000 ) ;
#6360=DIRECTION ( 'NONE',  ( 1.000000000000000000, 0.000000000000000000, -0.000000000000000000 ) ) ;
#6368=CARTESIAN_POINT ( 'NONE',  ( -107.5926225674731853, 102.8748711238780373, 20.00000000000000355 ) ) ;
#6398=LINE ( 'NONE', #15189, #1564 ) ;
#6428=VERTEX_POINT ( 'NONE', #10800 ) ;
#6454=ORIENTED_EDGE ( 'NONE', *, *, #1081, .T. ) ;
#6469=EDGE_LOOP ( 'NONE', ( #14425, #16674, #4695, #15512 ) ) ;
#6496=CARTESIAN_POINT ( 'NONE',  ( -97.59262256747318531, 0.3328663868096687350, -25.00000000000000000 ) ) ;
#6507=DIRECTION ( 'NONE',  ( 1.000000000000000000, 2.062304371594500494E-16, -2.775557561562890858E-16 ) ) ;
#6512=EDGE_CURVE ( 'NONE', #961, #10265, #15839, .T. ) ;
#6596=DIRECTION ( 'NONE',  ( -2.062304371594500494E-16, 1.000000000000000000, -0.000000000000000000 ) ) ;
#6623=CARTESIAN_POINT ( 'NONE',  ( -92.59262256747321373, 106.8071537307723133, -25.00000000000000000 ) ) ;
#6637=EDGE_CURVE ( 'NONE', #162, #15245, #11555, .T. ) ;
#6649=EDGE_CURVE ( 'NONE', #11466, #12161, #3301, .T. ) ;
#6658=DIRECTION ( 'NONE',  ( 0.000000000000000000, 0.000000000000000000, 1.000000000000000000 ) ) ;
#6660=CIRCLE ( 'NONE', #17122, 4.000000000000003553 ) ;
#6697=AXIS2_PLACEMENT_3D ( 'NONE', #262, #14488, #3429 ) ;
#6731=DIRECTION ( 'NONE',  ( -0.7071067811865474617, 8.659560562354932858E-17, -0.7071067811865474617 ) ) ;
#6733=DIRECTION ( 'NONE',  ( 1.000000000000000000, 2.062304371594500740E-16, 0.000000000000000000 ) ) ;
#6743=LINE ( 'NONE', #5044, #9727 ) ;
#6766=EDGE_LOOP ( 'NONE', ( #13502, #13833, #4409, #8667 ) ) ;
#6769=ADVANCED_FACE ( 'NONE', ( #11825 ), #9106, .F. ) ;
#6770=CARTESIAN_POINT ( 'NONE',  ( -107.5926225674731711, 57.88796029049330372, 30.35917033480640370 ) ) ;
#6776=DIRECTION ( 'NONE',  ( 0.000000000000000000, 1.000000000000000000, 0.000000000000000000 ) ) ;
#6801=CARTESIAN_POINT ( 'NONE',  ( -92.59262256747319952, 57.88796029049330372, 26.35917033480641436 ) ) ;
#6832=DIRECTION ( 'NONE',  ( -2.062304371594500494E-16, 1.000000000000000000, -0.000000000000000000 ) ) ;
#6872=CYLINDRICAL_SURFACE ( 'NONE', #15270, 9.999999999999994671 ) ;
#6873=DIRECTION ( 'NONE',  ( 1.000000000000000000, 2.062304371594500494E-16, 0.000000000000000000 ) ) ;
#6894=AXIS2_PLACEMENT_3D ( 'NONE', #11026, #15131, #829 ) ;
#6910=ORIENTED_EDGE ( 'NONE', *, *, #16367, .T. ) ;
#6915=LINE ( 'NONE', #9815, #3142 ) ;
#6916=DIRECTION ( 'NONE',  ( -1.000000000000000000, -0.000000000000000000, -0.000000000000000000 ) ) ;
#6948=ORIENTED_EDGE ( 'NONE', *, *, #1401, .F. ) ;
#6949=CARTESIAN_POINT ( 'NONE',  ( -107.5926225674731853, 110.5691553257988460, 26.35917033480641436 ) ) ;
#6960=AXIS2_PLACEMENT_3D ( 'NONE', #12101, #780, #2351 ) ;
#6963=DIRECTION ( 'NONE',  ( 1.000000000000000000, 2.062304371594500494E-16, 0.000000000000000000 ) ) ;
#6965=ORIENTED_EDGE ( 'NONE', *, *, #17958, .F. ) ;
#6968=EDGE_LOOP ( 'NONE', ( #9033, #15562, #7945, #621 ) ) ;
#6971=FACE_OUTER_BOUND ( 'NONE', #11554, .T. ) ;
#6983=DIRECTION ( 'NONE',  ( 0.000000000000000000, 0.000000000000000000, 1.000000000000000000 ) ) ;
#7010=PRODUCT_DEFINITION_FORMATION_WITH_SPECIFIED_SOURCE ( 'ANY', '', #13410, .NOT_KNOWN. ) ;
#7043=VECTOR ( 'NONE', #2968, 1000.000000000000000 ) ;
#7057=AXIS2_PLACEMENT_3D ( 'NONE', #7556, #6507, #18321 ) ;
#7061=VERTEX_POINT ( 'NONE', #5716 ) ;
#7063=VERTEX_POINT ( 'NONE', #2736 ) ;
#7074=DIRECTION ( 'NONE',  ( 0.000000000000000000, 1.000000000000000000, 0.000000000000000000 ) ) ;
#7081=ORIENTED_EDGE ( 'NONE', *, *, #1401, .T. ) ;
#7131=ADVANCED_FACE ( 'NONE', ( #3360 ), #6301, .F. ) ;
#7139=VECTOR ( 'NONE', #6832, 1000.000000000000000 ) ;
#7160=DIRECTION ( 'NONE',  ( -1.000000000000000000, -0.000000000000000000, -0.000000000000000000 ) ) ;
#7183=LINE ( 'NONE', #17003, #13160 ) ;
#7190=ORIENTED_EDGE ( 'NONE', *, *, #2184, .F. ) ;
#7206=CARTESIAN_POINT ( 'NONE',  ( -107.5676225674731654, 57.88796029049330372, 26.35917033480641436 ) ) ;
#7214=ADVANCED_FACE ( 'NONE', ( #6158 ), #14595, .F. ) ;
#7241=DIRECTION ( 'NONE',  ( -1.000000000000000000, -0.000000000000000000, -0.000000000000000000 ) ) ;
#7271=CARTESIAN_POINT ( 'NONE',  ( -97.59262256747319952, 57.88796029049330372, -26.35917033480641436 ) ) ;
#7272=DIRECTION ( 'NONE',  ( 0.000000000000000000, 0.000000000000000000, -1.000000000000000000 ) ) ;
#7277=VECTOR ( 'NONE', #17828, 1000.000000000000000 ) ;
#7289=CLOSED_SHELL ( 'NONE', ( #17953, #3114, #16922, #8850, #10766, #5368, #3258, #6769, #9973, #5325, #4034, #15212, #9051, #16013, #14239, #17492, #3908, #12391, #4435, #4023, #9498, #7131, #14831, #14301, #18448, #13053, #10287, #13152, #1342, #15465, #16678, #17062, #16199, #8325, #7445, #5929, #17815, #16962, #7214 ) ) ;
#7333=CARTESIAN_POINT ( 'NONE',  ( -102.5926225674731569, 65.58224449241410525, -20.00000000000000355 ) ) ;
#7344=EDGE_CURVE ( 'NONE', #7683, #857, #1276, .T. ) ;
#7348=CARTESIAN_POINT ( 'NONE',  ( -107.5926225674732137, 117.8748711238780373, 35.00000000000000000 ) ) ;
#7358=LINE ( 'NONE', #5923, #5777 ) ;
#7367=DIRECTION ( 'NONE',  ( 1.000000000000000000, 2.062304371594500494E-16, -2.775557561562890858E-16 ) ) ;
#7395=DIRECTION ( 'NONE',  ( 1.000000000000000000, 2.062304371594500740E-16, -0.000000000000000000 ) ) ;
#7407=CARTESIAN_POINT ( 'NONE',  ( -97.59262256747319952, 106.8071537307723133, 25.00000000000000000 ) ) ;
#7409=LINE ( 'NONE', #11625, #17103 ) ;
#7423=AXIS2_PLACEMENT_3D ( 'NONE', #15351, #8330, #14045 ) ;
#7440=DIRECTION ( 'NONE',  ( 0.000000000000000000, 1.734723475976811433E-15, 1.000000000000000000 ) ) ;
#7445=ADVANCED_FACE ( 'NONE', ( #607 ), #13338, .F. ) ;
#7458=EDGE_LOOP ( 'NONE', ( #9200, #10439, #13484, #7735 ) ) ;
#7488=DIRECTION ( 'NONE',  ( -1.000000000000000000, -2.062304371594500494E-16, 2.775557561562890858E-16 ) ) ;
#7495=ORIENTED_EDGE ( 'NONE', *, *, #7904, .F. ) ;
#7502=LINE ( 'NONE', #8911, #12323 ) ;
#7508=DIRECTION ( 'NONE',  ( 1.000000000000000000, 2.062304371594500740E-16, -0.000000000000000000 ) ) ;
#7510=AXIS2_PLACEMENT_3D ( 'NONE', #2562, #8262, #15730 ) ;
#7515=DIRECTION ( 'NONE',  ( -2.062304371594500494E-16, 1.000000000000000000, -0.000000000000000000 ) ) ;
#7518=APPLICATION_CONTEXT ( 'automotive_design' ) ;
#7532=DIRECTION ( 'NONE',  ( -1.000000000000000000, 0.000000000000000000, 0.000000000000000000 ) ) ;
#7533=CARTESIAN_POINT ( 'NONE',  ( -107.5926225674732137, 117.8748711238780373, 35.00000000000000000 ) ) ;
#7534=ORIENTED_EDGE ( 'NONE', *, *, #6512, .T. ) ;
#7556=CARTESIAN_POINT ( 'NONE',  ( -97.59262256747319952, 110.5691553257988460, 26.35917033480641436 ) ) ;
#7557=CARTESIAN_POINT ( 'NONE',  ( -107.5926225674731853, 110.5691553257988460, -22.33417033480641223 ) ) ;
#7562=EDGE_CURVE ( 'NONE', #15190, #7061, #16124, .T. ) ;
#7568=DIRECTION ( 'NONE',  ( 1.000000000000000000, -0.000000000000000000, -0.000000000000000000 ) ) ;
#7585=FACE_OUTER_BOUND ( 'NONE', #2032, .T. ) ;
#7589=CARTESIAN_POINT ( 'NONE',  ( -107.5926225674731711, 65.58224449241410525, 20.00000000000000355 ) ) ;
#7596=EDGE_CURVE ( 'NONE', #9962, #4700, #3051, .T. ) ;
#7604=VECTOR ( 'NONE', #2287, 1000.000000000000000 ) ;
#7625=EDGE_LOOP ( 'NONE', ( #3994, #5071, #12126, #1988 ) ) ;
#7645=DIRECTION ( 'NONE',  ( -1.000000000000000000, 0.000000000000000000, 0.000000000000000000 ) ) ;
#7650=CARTESIAN_POINT ( 'NONE',  ( -107.5926225674731711, 57.88796029049330372, -30.38417033480641294 ) ) ;
#7671=DIRECTION ( 'NONE',  ( 0.000000000000000000, 0.000000000000000000, 1.000000000000000000 ) ) ;
#7672=ORIENTED_EDGE ( 'NONE', *, *, #10618, .F. ) ;
#7683=VERTEX_POINT ( 'NONE', #9398 ) ;
#7689=FACE_OUTER_BOUND ( 'NONE', #16927, .T. ) ;
#7693=FACE_OUTER_BOUND ( 'NONE', #214, .T. ) ;
#7722=DIRECTION ( 'NONE',  ( -1.000000000000000000, -0.000000000000000000, -0.000000000000000000 ) ) ;
#7729=ORIENTED_EDGE ( 'NONE', *, *, #11909, .F. ) ;
#7735=ORIENTED_EDGE ( 'NONE', *, *, #7562, .F. ) ;
#7755=EDGE_LOOP ( 'NONE', ( #16397, #8802, #15686, #15603, #4156, #10580 ) ) ;
#7761=LINE ( 'NONE', #7589, #14343 ) ;
#7764=EDGE_CURVE ( 'NONE', #15245, #17316, #15907, .T. ) ;
#7778=DIRECTION ( 'NONE',  ( 0.000000000000000000, 0.000000000000000000, 1.000000000000000000 ) ) ;
#7789=EDGE_LOOP ( 'NONE', ( #49, #3640, #16748, #990 ) ) ;
#7800=LINE ( 'NONE', #7978, #5810 ) ;
#7807=DIRECTION ( 'NONE',  ( 0.000000000000000000, 3.469446951953617344E-15, 1.000000000000000000 ) ) ;
#7814=DIRECTION ( 'NONE',  ( 0.000000000000000000, 0.000000000000000000, 1.000000000000000000 ) ) ;
#7815=AXIS2_PLACEMENT_3D ( 'NONE', #755, #10472, #7671 ) ;
#7819=DIRECTION ( 'NONE',  ( 0.000000000000000000, 0.000000000000000000, 1.000000000000000000 ) ) ;
#7821=AXIS2_PLACEMENT_3D ( 'NONE', #7271, #17443, #7440 ) ;
#7825=DIRECTION ( 'NONE',  ( 0.000000000000000000, 1.000000000000000000, 0.000000000000000000 ) ) ;
#7832=DIRECTION ( 'NONE',  ( -1.000000000000000000, -2.062304371594500740E-16, -0.000000000000000000 ) ) ;
#7834=CARTESIAN_POINT ( 'NONE',  ( -97.59262256747321373, 110.5691553257988460, -26.35917033480641436 ) ) ;
#7845=LINE ( 'NONE', #9526, #12960 ) ;
#7857=AXIS2_PLACEMENT_3D ( 'NONE', #12909, #3327, #13005 ) ;
#7880=DIRECTION ( 'NONE',  ( -1.000000000000000000, -2.062304371594500494E-16, -0.000000000000000000 ) ) ;
#7888=VECTOR ( 'NONE', #11461, 1000.000000000000000 ) ;
#7895=AXIS2_PLACEMENT_3D ( 'NONE', #7834, #11951, #10652 ) ;
#7900=EDGE_CURVE ( 'NONE', #3688, #9785, #9937, .T. ) ;
#7904=EDGE_CURVE ( 'NONE', #7063, #15333, #7502, .T. ) ;
#7919=ORIENTED_EDGE ( 'NONE', *, *, #18069, .F. ) ;
#7924=CARTESIAN_POINT ( 'NONE',  ( -107.5926225674731711, 57.88796029049330372, -22.35917033480642502 ) ) ;
#7928=ORIENTED_EDGE ( 'NONE', *, *, #47, .T. ) ;
#7929=CIRCLE ( 'NONE', #18402, 9.999999999999994671 ) ;
#7930=DIRECTION ( 'NONE',  ( -2.062304371594500494E-16, 1.000000000000000000, 0.000000000000000000 ) ) ;
#7945=ORIENTED_EDGE ( 'NONE', *, *, #11111, .F. ) ;
#7946=DIRECTION ( 'NONE',  ( -1.000000000000000000, -0.000000000000000000, -0.000000000000000000 ) ) ;
#7954=CARTESIAN_POINT ( 'NONE',  ( -107.5926225674732137, 117.8748711238780373, -25.00000000000000000 ) ) ;
#7978=CARTESIAN_POINT ( 'NONE',  ( -107.5926225674731853, 50.58224449241411236, -25.00000000000000000 ) ) ;
#7992=EDGE_CURVE ( 'NONE', #16431, #3688, #7409, .T. ) ;
#8026=DIRECTION ( 'NONE',  ( -1.000000000000000000, -0.000000000000000000, -0.000000000000000000 ) ) ;
#8031=DIRECTION ( 'NONE',  ( 1.000000000000000000, 2.062304371594500494E-16, 0.000000000000000000 ) ) ;
#8042=VERTEX_POINT ( 'NONE', #6263 ) ;
#8073=DIRECTION ( 'NONE',  ( -1.000000000000000000, -0.000000000000000000, -0.000000000000000000 ) ) ;
#8088=ORIENTED_EDGE ( 'NONE', *, *, #8488, .T. ) ;
#8122=DIRECTION ( 'NONE',  ( -2.062304371594500494E-16, 1.000000000000000000, -0.000000000000000000 ) ) ;
#8157=AXIS2_PLACEMENT_3D ( 'NONE', #15199, #7722, #7819 ) ;
#8159=DIRECTION ( 'NONE',  ( 0.000000000000000000, 0.000000000000000000, 1.000000000000000000 ) ) ;
#8195=AXIS2_PLACEMENT_3D ( 'NONE', #9788, #18488, #6983 ) ;
#8201=EDGE_LOOP ( 'NONE', ( #4854, #6123, #735, #16880, #12907, #2335 ) ) ;
#8223=EDGE_CURVE ( 'NONE', #2867, #11561, #17700, .T. ) ;
#8224=CARTESIAN_POINT ( 'NONE',  ( -92.59262256747318531, 0.3328663868096687350, 25.00000000000000000 ) ) ;
#8245=LINE ( 'NONE', #12368, #7139 ) ;
#8253=DIRECTION ( 'NONE',  ( -1.000000000000000000, -2.062304371594500494E-16, -0.000000000000000000 ) ) ;
#8262=DIRECTION ( 'NONE',  ( 1.000000000000000000, 2.062304371594500740E-16, 0.000000000000000000 ) ) ;
#8277=VERTEX_POINT ( 'NONE', #13770 ) ;
#8284=CARTESIAN_POINT ( 'NONE',  ( -92.59262256747319952, 57.88796029049330372, -30.35917033480640370 ) ) ;
#8296=CARTESIAN_POINT ( 'NONE',  ( -107.5926225674731711, 65.58224449241410525, 20.00000000000000355 ) ) ;
#8305=EDGE_LOOP ( 'NONE', ( #6965, #15966, #9908, #8607, #12174 ) ) ;
#8316=LINE ( 'NONE', #17009, #15082 ) ;
#8322=FACE_OUTER_BOUND ( 'NONE', #5066, .T. ) ;
#8325=ADVANCED_FACE ( 'NONE', ( #5153 ), #15157, .F. ) ;
#8330=DIRECTION ( 'NONE',  ( 0.000000000000000000, 0.000000000000000000, 1.000000000000000000 ) ) ;
#8353=DIRECTION ( 'NONE',  ( -1.000000000000000000, -0.000000000000000000, -0.000000000000000000 ) ) ;
#8381=ORIENTED_EDGE ( 'NONE', *, *, #17445, .F. ) ;
#8389=CIRCLE ( 'NONE', #3006, 3.999999999999996447 ) ;
#8404=VERTEX_POINT ( 'NONE', #1575 ) ;
#8417=CARTESIAN_POINT ( 'NONE',  ( -97.59262256747317110, 0.3328663868096687350, 25.00000000000000000 ) ) ;
#8436=CIRCLE ( 'NONE', #5428, 4.025000000000000355 ) ;
#8451=EDGE_LOOP ( 'NONE', ( #3092, #7081, #17446, #16943, #15658, #12771 ) ) ;
#8488=EDGE_CURVE ( 'NONE', #15333, #14280, #13440, .T. ) ;
#8497=VECTOR ( 'NONE', #6596, 1000.000000000000000 ) ;
#8515=AXIS2_PLACEMENT_3D ( 'NONE', #10680, #9099, #7778 ) ;
#8525=AXIS2_PLACEMENT_3D ( 'NONE', #5658, #9882, #1099 ) ;
#8550=ORIENTED_EDGE ( 'NONE', *, *, #14091, .F. ) ;
#8568=FACE_OUTER_BOUND ( 'NONE', #10164, .T. ) ;
#8607=ORIENTED_EDGE ( 'NONE', *, *, #14235, .F. ) ;
#8648=DIRECTION ( 'NONE',  ( 1.000000000000000000, 2.062304371594500494E-16, 0.000000000000000000 ) ) ;
#8663=CARTESIAN_POINT ( 'NONE',  ( -92.59262256747321373, 114.3311569208253786, -25.00000000000000000 ) ) ;
#8665=VECTOR ( 'NONE', #16756, 1000.000000000000114 ) ;
#8667=ORIENTED_EDGE ( 'NONE', *, *, #6637, .F. ) ;
#8681=CIRCLE ( 'NONE', #6894, 3.999999999999989786 ) ;
#8727=CARTESIAN_POINT ( 'NONE',  ( -107.5926225674732137, 117.8748711238780373, -25.00000000000000000 ) ) ;
#8738=APPLICATION_CONTEXT ( 'automotive_design' ) ;
#8769=AXIS2_PLACEMENT_3D ( 'NONE', #5513, #6916, #16924 ) ;
#8802=ORIENTED_EDGE ( 'NONE', *, *, #16810, .T. ) ;
#8850=ADVANCED_FACE ( 'NONE', ( #14815 ), #16308, .F. ) ;
#8864=DIRECTION ( 'NONE',  ( 2.062304371594500247E-16, -1.000000000000000000, 0.000000000000000000 ) ) ;
#8875=( LENGTH_UNIT ( ) NAMED_UNIT ( * ) SI_UNIT ( .MILLI., .METRE. ) );
#8911=CARTESIAN_POINT ( 'NONE',  ( -107.5926225674731711, 61.64996188551983636, 25.00000000000000000 ) ) ;
#8912=EDGE_CURVE ( 'NONE', #2797, #11561, #13793, .T. ) ;
#8913=ORIENTED_EDGE ( 'NONE', *, *, #11144, .F. ) ;
#8921=ORIENTED_EDGE ( 'NONE', *, *, #13582, .F. ) ;
#8946=CARTESIAN_POINT ( 'NONE',  ( -107.5926225674731853, 102.8748711238780373, -20.00000000000000355 ) ) ;
#8961=DIRECTION ( 'NONE',  ( 1.000000000000000000, 0.000000000000000000, 0.000000000000000000 ) ) ;
#8964=ORIENTED_EDGE ( 'NONE', *, *, #10071, .T. ) ;
#8993=CARTESIAN_POINT ( 'NONE',  ( -107.5926225674731711, 57.88796029049330372, 26.35917033480641436 ) ) ;
#9017=DIRECTION ( 'NONE',  ( 0.000000000000000000, 1.000000000000000000, 0.000000000000000000 ) ) ;
#9025=VECTOR ( 'NONE', #9635, 1000.000000000000000 ) ;
#9033=ORIENTED_EDGE ( 'NONE', *, *, #16836, .T. ) ;
#9038=LINE ( 'NONE', #7533, #13511 ) ;
#9051=ADVANCED_FACE ( 'NONE', ( #7689 ), #5058, .F. ) ;
#9078=DIRECTION ( 'NONE',  ( 0.000000000000000000, 1.000000000000000000, 0.000000000000000000 ) ) ;
#9090=VECTOR ( 'NONE', #15853, 1000.000000000000000 ) ;
#9099=DIRECTION ( 'NONE',  ( -1.000000000000000000, -0.000000000000000000, -0.000000000000000000 ) ) ;
#9106=CYLINDRICAL_SURFACE ( 'NONE', #1536, 3.999999999999989786 ) ;
#9114=ORIENTED_EDGE ( 'NONE', *, *, #1920, .F. ) ;
#9130=DIRECTION ( 'NONE',  ( 7.442644330182800165E-16, -1.000000000000000000, 0.000000000000000000 ) ) ;
#9136=VERTEX_POINT ( 'NONE', #10872 ) ;
#9165=VERTEX_POINT ( 'NONE', #12475 ) ;
#9172=CARTESIAN_POINT ( 'NONE',  ( -107.5926225674732137, 107.8748711238780373, -35.00000000000000000 ) ) ;
#9180=LINE ( 'NONE', #7954, #9358 ) ;
#9187=EDGE_LOOP ( 'NONE', ( #2134, #16031, #8381, #10981 ) ) ;
#9200=ORIENTED_EDGE ( 'NONE', *, *, #2518, .F. ) ;
#9240=ORIENTED_EDGE ( 'NONE', *, *, #10870, .T. ) ;
#9241=DIRECTION ( 'NONE',  ( -0.7071067811864494290, 0.000000000000000000, 0.7071067811866454944 ) ) ;
#9244=EDGE_CURVE ( 'NONE', #827, #16099, #1549, .T. ) ;
#9249=CARTESIAN_POINT ( 'NONE',  ( -107.5926225674731711, 57.88796029049330372, -22.33417033480641223 ) ) ;
#9255=EDGE_CURVE ( 'NONE', #8042, #5082, #8436, .T. ) ;
#9288=DIRECTION ( 'NONE',  ( 1.000000000000000000, 2.062304371594500494E-16, 0.000000000000000000 ) ) ;
#9293=EDGE_LOOP ( 'NONE', ( #17949, #1334 ) ) ;
#9298=VECTOR ( 'NONE', #2762, 1000.000000000000000 ) ;
#9305=ORIENTED_EDGE ( 'NONE', *, *, #4271, .F. ) ;
#9314=CIRCLE ( 'NONE', #15882, 3.999999999999989786 ) ;
#9342=ORIENTED_EDGE ( 'NONE', *, *, #4548, .T. ) ;
#9343=CIRCLE ( 'NONE', #12331, 9.999999999999994671 ) ;
#9345=CARTESIAN_POINT ( 'NONE',  ( -102.5926225674731853, 102.8748711238780373, 20.00000000000000355 ) ) ;
#9348=DIRECTION ( 'NONE',  ( 1.000000000000000000, 2.062304371594500494E-16, 0.000000000000000000 ) ) ;
#9352=CARTESIAN_POINT ( 'NONE',  ( -102.5926225674731853, 102.8748711238780373, 20.00000000000000355 ) ) ;
#9358=VECTOR ( 'NONE', #10475, 1000.000000000000000 ) ;
#9378=DIRECTION ( 'NONE',  ( 0.000000000000000000, 0.000000000000000000, 1.000000000000000000 ) ) ;
#9379=CARTESIAN_POINT ( 'NONE',  ( -107.5926225674731853, 107.8748711238780373, -25.00000000000000000 ) ) ;
#9387=PLANE ( 'NONE',  #2030 ) ;
#9398=CARTESIAN_POINT ( 'NONE',  ( -97.59262256747319952, 61.64996188551983636, -25.00000000000000000 ) ) ;
#9401=VECTOR ( 'NONE', #16772, 1000.000000000000000 ) ;
#9461=PLANE ( 'NONE',  #5452 ) ;
#9464=FACE_OUTER_BOUND ( 'NONE', #17773, .T. ) ;
#9470=CARTESIAN_POINT ( 'NONE',  ( -97.59262256747318531, 54.12595869546677818, 25.00000000000000000 ) ) ;
#9498=ADVANCED_FACE ( 'NONE', ( #7585 ), #13567, .F. ) ;
#9520=ORIENTED_EDGE ( 'NONE', *, *, #16462, .F. ) ;
#9526=CARTESIAN_POINT ( 'NONE',  ( -92.59262256747318531, 0.3328663868096687350, 25.00000000000000000 ) ) ;
#9635=DIRECTION ( 'NONE',  ( -1.000000000000000000, -2.062304371594500247E-16, -0.000000000000000000 ) ) ;
#9646=ORIENTED_EDGE ( 'NONE', *, *, #7764, .T. ) ;
#9685=CARTESIAN_POINT ( 'NONE',  ( -92.59262256747321373, 110.5691553257988460, -26.35917033480641436 ) ) ;
#9703=EDGE_CURVE ( 'NONE', #18220, #12020, #4119, .T. ) ;
#9727=VECTOR ( 'NONE', #13951, 1000.000000000000000 ) ;
#9756=DIRECTION ( 'NONE',  ( -1.000000000000000000, -0.000000000000000000, -0.000000000000000000 ) ) ;
#9766=CARTESIAN_POINT ( 'NONE',  ( -107.5926225674731853, 110.5691553257988460, -30.38417033480641294 ) ) ;
#9768=EDGE_CURVE ( 'NONE', #3038, #14123, #5605, .T. ) ;
#9781=DIRECTION ( 'NONE',  ( 1.000000000000000000, 2.062304371594500494E-16, 0.000000000000000000 ) ) ;
#9785=VERTEX_POINT ( 'NONE', #10183 ) ;
#9788=CARTESIAN_POINT ( 'NONE',  ( -107.5926225674731853, 110.5691553257988460, -26.35917033480641436 ) ) ;
#9815=CARTESIAN_POINT ( 'NONE',  ( -107.5926225674731853, 110.5691553257988460, -22.35917033480641791 ) ) ;
#9816=DIRECTION ( 'NONE',  ( -1.000000000000000000, -0.000000000000000000, -0.000000000000000000 ) ) ;
#9822=DIRECTION ( 'NONE',  ( -1.000000000000000000, -0.000000000000000000, -0.000000000000000000 ) ) ;
#9826=DIRECTION ( 'NONE',  ( 0.000000000000000000, 0.000000000000000000, 1.000000000000000000 ) ) ;
#9856=AXIS2_PLACEMENT_3D ( 'NONE', #7348, #2866, #15939 ) ;
#9870=CARTESIAN_POINT ( 'NONE',  ( -107.5926225674731711, 54.12595869546677818, 25.00000000000000000 ) ) ;
#9872=CARTESIAN_POINT ( 'NONE',  ( -92.59262256747318531, -1.909541702982995504E-14, 0.000000000000000000 ) ) ;
#9880=ORIENTED_EDGE ( 'NONE', *, *, #2293, .T. ) ;
#9882=DIRECTION ( 'NONE',  ( 1.000000000000000000, 2.062304371594500494E-16, 0.000000000000000000 ) ) ;
#9908=ORIENTED_EDGE ( 'NONE', *, *, #11457, .F. ) ;
#9912=AXIS2_PLACEMENT_3D ( 'NONE', #8993, #14864, #16276 ) ;
#9935=CARTESIAN_POINT ( 'NONE',  ( -92.59262256747318531, 0.3328663868096687350, -25.00000000000000000 ) ) ;
#9937=CIRCLE ( 'NONE', #10236, 4.000000000000003553 ) ;
#9955=CIRCLE ( 'NONE', #4550, 3.999999999999989786 ) ;
#9960=ORIENTED_EDGE ( 'NONE', *, *, #13618, .T. ) ;
#9962=VERTEX_POINT ( 'NONE', #5745 ) ;
#9965=EDGE_LOOP ( 'NONE', ( #1336, #13361 ) ) ;
#9973=ADVANCED_FACE ( 'NONE', ( #8568 ), #14085, .T. ) ;
#9981=EDGE_CURVE ( 'NONE', #2087, #3821, #9955, .T. ) ;
#10071=EDGE_CURVE ( 'NONE', #10167, #11961, #4259, .T. ) ;
#10097=EDGE_LOOP ( 'NONE', ( #1997, #15663, #18369, #6018 ) ) ;
#10107=EDGE_LOOP ( 'NONE', ( #1977, #2196, #10286, #1372, #7919, #18093, #4791, #8913, #12158, #16065 ) ) ;
#10131=LINE ( 'NONE', #217, #7888 ) ;
#10160=CARTESIAN_POINT ( 'NONE',  ( -102.5926225674731569, 65.58224449241410525, -20.00000000000000355 ) ) ;
#10164=EDGE_LOOP ( 'NONE', ( #9880, #3154, #15011, #11695, #12319, #17745, #18451, #8088, #12298, #1504 ) ) ;
#10167=VERTEX_POINT ( 'NONE', #12972 ) ;
#10170=CONICAL_SURFACE ( 'NONE', #12260, 4.025000000000000355, 0.7853981633975870569 ) ;
#10183=CARTESIAN_POINT ( 'NONE',  ( -107.5676225674731938, 110.5691553257988460, 30.35917033480641791 ) ) ;
#10193=ORIENTED_EDGE ( 'NONE', *, *, #17381, .F. ) ;
#10202=CARTESIAN_POINT ( 'NONE',  ( -102.5926225674731853, 102.8748711238780373, 20.00000000000000355 ) ) ;
#10227=ORIENTED_EDGE ( 'NONE', *, *, #10660, .T. ) ;
#10236=AXIS2_PLACEMENT_3D ( 'NONE', #14529, #7241, #17320 ) ;
#10265=VERTEX_POINT ( 'NONE', #9470 ) ;
#10276=LINE ( 'NONE', #7650, #1657 ) ;
#10286=ORIENTED_EDGE ( 'NONE', *, *, #10071, .F. ) ;
#10287=ADVANCED_FACE ( 'NONE', ( #17796 ), #682, .F. ) ;
#10291=EDGE_CURVE ( 'NONE', #17316, #14280, #13527, .T. ) ;
#10294=CIRCLE ( 'NONE', #5819, 4.000000000000003553 ) ;
#10315=AXIS2_PLACEMENT_3D ( 'NONE', #3603, #623, #2210 ) ;
#10366=LINE ( 'NONE', #11770, #16412 ) ;
#10373=DIRECTION ( 'NONE',  ( -1.000000000000000000, -0.000000000000000000, -0.000000000000000000 ) ) ;
#10376=ORIENTED_EDGE ( 'NONE', *, *, #9703, .T. ) ;
#10396=EDGE_CURVE ( 'NONE', #11747, #11084, #13879, .T. ) ;
#10404=AXIS2_PLACEMENT_3D ( 'NONE', #10787, #12107, #15085 ) ;
#10439=ORIENTED_EDGE ( 'NONE', *, *, #17822, .T. ) ;
#10461=VERTEX_POINT ( 'NONE', #15464 ) ;
#10465=DIRECTION ( 'NONE',  ( 0.000000000000000000, 0.000000000000000000, 1.000000000000000000 ) ) ;
#10466=DIRECTION ( 'NONE',  ( -1.000000000000000000, -2.062304371594500740E-16, 0.000000000000000000 ) ) ;
#10472=DIRECTION ( 'NONE',  ( -1.000000000000000000, -0.000000000000000000, -0.000000000000000000 ) ) ;
#10475=DIRECTION ( 'NONE',  ( -1.000000000000000000, -2.062304371594500740E-16, -0.000000000000000000 ) ) ;
#10496=AXIS2_PLACEMENT_3D ( 'NONE', #17975, #15263, #94 ) ;
#10499=EDGE_CURVE ( 'NONE', #11807, #13603, #16513, .T. ) ;
#10509=CIRCLE ( 'NONE', #2456, 3.999999999999989786 ) ;
#10518=DIRECTION ( 'NONE',  ( 1.000000000000000000, 0.000000000000000000, 0.000000000000000000 ) ) ;
#10548=CARTESIAN_POINT ( 'NONE',  ( -107.5676225674731938, 110.5691553257988460, -22.35917033480641081 ) ) ;
#10559=CARTESIAN_POINT ( 'NONE',  ( -92.59262256747321373, 117.8748711238780515, 25.00000000000000000 ) ) ;
#10566=DIRECTION ( 'NONE',  ( -1.000000000000000000, -0.000000000000000000, -0.000000000000000000 ) ) ;
#10580=ORIENTED_EDGE ( 'NONE', *, *, #15206, .T. ) ;
#10618=EDGE_CURVE ( 'NONE', #8277, #1119, #11541, .T. ) ;
#10625=ORIENTED_EDGE ( 'NONE', *, *, #14423, .T. ) ;
#10627=AXIS2_PLACEMENT_3D ( 'NONE', #12152, #17839, #2224 ) ;
#10633=ORIENTED_EDGE ( 'NONE', *, *, #7344, .F. ) ;
#10647=LINE ( 'NONE', #909, #4249 ) ;
#10648=ORIENTED_EDGE ( 'NONE', *, *, #1140, .T. ) ;
#10652=DIRECTION ( 'NONE',  ( 0.000000000000000000, 6.938893903907234689E-15, 1.000000000000000000 ) ) ;
#10660=EDGE_CURVE ( 'NONE', #1119, #3000, #9180, .T. ) ;
#10665=CARTESIAN_POINT ( 'NONE',  ( -97.59262256747318531, 57.88796029049330372, 26.35917033480641436 ) ) ;
#10680=CARTESIAN_POINT ( 'NONE',  ( -107.5926225674731853, 110.5691553257988460, 26.35917033480641436 ) ) ;
#10715=CARTESIAN_POINT ( 'NONE',  ( -107.5926225674731853, 50.58224449241411236, 25.00000000000000000 ) ) ;
#10760=EDGE_CURVE ( 'NONE', #16099, #827, #6660, .T. ) ;
#10763=MECHANICAL_DESIGN_GEOMETRIC_PRESENTATION_REPRESENTATION('',(#14077),#12586);
#10766=ADVANCED_FACE ( 'NONE', ( #2017 ), #5766, .F. ) ;
#10787=CARTESIAN_POINT ( 'NONE',  ( -107.5926225674731711, 57.88796029049330372, -26.35917033480641436 ) ) ;
#10792=CARTESIAN_POINT ( 'NONE',  ( -107.5676225674731654, 57.88796029049330372, 30.35917033480641081 ) ) ;
#10800=CARTESIAN_POINT ( 'NONE',  ( -107.5676225674731654, 57.88796029049330372, -30.35917033480641081 ) ) ;
#10810=AXIS2_PLACEMENT_3D ( 'NONE', #16293, #676, #4771 ) ;
#10847=CARTESIAN_POINT ( 'NONE',  ( -92.59262256747319952, 57.88796029049330372, 30.35917033480640370 ) ) ;
#10870=EDGE_CURVE ( 'NONE', #14275, #5132, #11937, .T. ) ;
#10871=DIRECTION ( 'NONE',  ( 0.000000000000000000, 0.000000000000000000, 1.000000000000000000 ) ) ;
#10872=CARTESIAN_POINT ( 'NONE',  ( -107.5926225674732137, 107.8748711238780373, 35.00000000000000000 ) ) ;
#10881=ORIENTED_EDGE ( 'NONE', *, *, #7992, .F. ) ;
#10897=ORIENTED_EDGE ( 'NONE', *, *, #14423, .F. ) ;
#10947=LINE ( 'NONE', #11319, #1075 ) ;
#10951=DIRECTION ( 'NONE',  ( -1.000000000000000000, -2.062304371594500247E-16, 0.000000000000000000 ) ) ;
#10969=DIRECTION ( 'NONE',  ( -1.000000000000000000, -0.000000000000000000, -0.000000000000000000 ) ) ;
#10981=ORIENTED_EDGE ( 'NONE', *, *, #16926, .F. ) ;
#11012=ORIENTED_EDGE ( 'NONE', *, *, #7900, .F. ) ;
#11016=DIRECTION ( 'NONE',  ( 1.000000000000000000, 2.062304371594500494E-16, 0.000000000000000000 ) ) ;
#11026=CARTESIAN_POINT ( 'NONE',  ( -97.59262256747319952, 57.88796029049330372, -26.35917033480641436 ) ) ;
#11040=PRODUCT_DEFINITION_SHAPE ( 'NONE', 'NONE',  #4980 ) ;
#11069=ORIENTED_EDGE ( 'NONE', *, *, #3063, .F. ) ;
#11084=VERTEX_POINT ( 'NONE', #6013 ) ;
#11111=EDGE_CURVE ( 'NONE', #3038, #18456, #15770, .T. ) ;
#11115=AXIS2_PLACEMENT_3D ( 'NONE', #1779, #7488, #17571 ) ;
#11116=CARTESIAN_POINT ( 'NONE',  ( -92.59262256747318531, 0.3328663868096687350, -25.00000000000000000 ) ) ;
#11144=EDGE_CURVE ( 'NONE', #13494, #2247, #7358, .T. ) ;
#11148=AXIS2_PLACEMENT_3D ( 'NONE', #4225, #11157, #15738 ) ;
#11157=DIRECTION ( 'NONE',  ( -1.000000000000000000, -0.000000000000000000, -0.000000000000000000 ) ) ;
#11163=CIRCLE ( 'NONE', #7857, 3.999999999999989786 ) ;
#11216=FACE_OUTER_BOUND ( 'NONE', #7458, .T. ) ;
#11237=CIRCLE ( 'NONE', #7057, 3.999999999999996447 ) ;
#11251=ORIENTED_EDGE ( 'NONE', *, *, #2375, .T. ) ;
#11253=CARTESIAN_POINT ( 'NONE',  ( -97.59262256747321373, 114.3311569208253786, -25.00000000000000000 ) ) ;
#11257=EDGE_CURVE ( 'NONE', #8404, #13480, #16441, .T. ) ;
#11262=CARTESIAN_POINT ( 'NONE',  ( -107.5926225674731711, 57.88796029049330372, 26.35917033480641436 ) ) ;
#11269=DIRECTION ( 'NONE',  ( -1.000000000000000000, -0.000000000000000000, -0.000000000000000000 ) ) ;
#11285=DIRECTION ( 'NONE',  ( 0.000000000000000000, 1.000000000000000000, 0.000000000000000000 ) ) ;
#11305=DIRECTION ( 'NONE',  ( -1.000000000000000000, 0.000000000000000000, 0.000000000000000000 ) ) ;
#11319=CARTESIAN_POINT ( 'NONE',  ( -107.5926225674731853, 110.5691553257988460, 22.33417033480641223 ) ) ;
#11320=LINE ( 'NONE', #4202, #3082 ) ;
#11328=ORIENTED_EDGE ( 'NONE', *, *, #7562, .T. ) ;
#11362=AXIS2_PLACEMENT_3D ( 'NONE', #14883, #18166, #10871 ) ;
#11381=VECTOR ( 'NONE', #16633, 1000.000000000000000 ) ;
#11383=VECTOR ( 'NONE', #7568, 1000.000000000000000 ) ;
#11406=VECTOR ( 'NONE', #15104, 1000.000000000000000 ) ;
#11411=DIRECTION ( 'NONE',  ( -0.7071067811865474617, 0.000000000000000000, 0.7071067811865474617 ) ) ;
#11457=EDGE_CURVE ( 'NONE', #16207, #18159, #1020, .T. ) ;
#11458=CIRCLE ( 'NONE', #16203, 3.999999999999989786 ) ;
#11461=DIRECTION ( 'NONE',  ( -2.062304371594500494E-16, 1.000000000000000000, -0.000000000000000000 ) ) ;
#11466=VERTEX_POINT ( 'NONE', #11768 ) ;
#11532=VECTOR ( 'NONE', #15479, 1000.000000000000000 ) ;
#11541=LINE ( 'NONE', #8727, #1314 ) ;
#11551=DIRECTION ( 'NONE',  ( -1.000000000000000000, -0.000000000000000000, -0.000000000000000000 ) ) ;
#11554=EDGE_LOOP ( 'NONE', ( #15697, #12324, #7672, #878, #9114 ) ) ;
#11555=LINE ( 'NONE', #16970, #9298 ) ;
#11561=VERTEX_POINT ( 'NONE', #2498 ) ;
#11563=ORIENTED_EDGE ( 'NONE', *, *, #3527, .F. ) ;
#11565=EDGE_CURVE ( 'NONE', #12447, #961, #17436, .T. ) ;
#11599=CARTESIAN_POINT ( 'NONE',  ( -107.5926225674731711, 57.88796029049330372, 26.35917033480641436 ) ) ;
#11600=ORIENTED_EDGE ( 'NONE', *, *, #159, .F. ) ;
#11610=FACE_OUTER_BOUND ( 'NONE', #18158, .T. ) ;
#11615=DIRECTION ( 'NONE',  ( 1.000000000000000000, 0.000000000000000000, -0.000000000000000000 ) ) ;
#11619=EDGE_LOOP ( 'NONE', ( #13862, #2543, #13224, #17590 ) ) ;
#11625=CARTESIAN_POINT ( 'NONE',  ( -107.5926225674731853, 110.5691553257988460, 22.35917033480641791 ) ) ;
#11690=LINE ( 'NONE', #10559, #11383 ) ;
#11695=ORIENTED_EDGE ( 'NONE', *, *, #159, .T. ) ;
#11731=VERTEX_POINT ( 'NONE', #2883 ) ;
#11738=ORIENTED_EDGE ( 'NONE', *, *, #7596, .F. ) ;
#11747=VERTEX_POINT ( 'NONE', #14289 ) ;
#11762=ORIENTED_EDGE ( 'NONE', *, *, #18331, .F. ) ;
#11768=CARTESIAN_POINT ( 'NONE',  ( -107.5926225674731853, 50.58224449241411236, 25.00000000000000000 ) ) ;
#11770=CARTESIAN_POINT ( 'NONE',  ( -102.5926225674731853, 102.8748711238780373, -20.00000000000000355 ) ) ;
#11783=ORIENTED_EDGE ( 'NONE', *, *, #1717, .F. ) ;
#11789=EDGE_CURVE ( 'NONE', #2130, #5246, #14479, .T. ) ;
#11792=VECTOR ( 'NONE', #10566, 1000.000000000000000 ) ;
#11807=VERTEX_POINT ( 'NONE', #14721 ) ;
#11813=VECTOR ( 'NONE', #9822, 1000.000000000000000 ) ;
#11816=ORIENTED_EDGE ( 'NONE', *, *, #2291, .F. ) ;
#11825=FACE_OUTER_BOUND ( 'NONE', #13112, .T. ) ;
#11827=LINE ( 'NONE', #17326, #2526 ) ;
#11866=DIRECTION ( 'NONE',  ( -2.062304371594500494E-16, 1.000000000000000000, 0.000000000000000000 ) ) ;
#11872=CARTESIAN_POINT ( 'NONE',  ( -102.5926225674731569, 65.58224449241410525, 20.00000000000000355 ) ) ;
#11874=LINE ( 'NONE', #7924, #16686 ) ;
#11909=EDGE_CURVE ( 'NONE', #16431, #162, #143, .T. ) ;
#11937=LINE ( 'NONE', #10715, #706 ) ;
#11951=DIRECTION ( 'NONE',  ( 1.000000000000000000, 2.062304371594500494E-16, -2.775557561562890858E-16 ) ) ;
#11957=VECTOR ( 'NONE', #9241, 1000.000000000000000 ) ;
#11961=VERTEX_POINT ( 'NONE', #2277 ) ;
#11988=ORIENTED_EDGE ( 'NONE', *, *, #6273, .F. ) ;
#12020=VERTEX_POINT ( 'NONE', #3498 ) ;
#12048=FACE_BOUND ( 'NONE', #12811, .T. ) ;
#12066=CARTESIAN_POINT ( 'NONE',  ( -107.5676225674731938, 110.5691553257988460, 26.35917033480641436 ) ) ;
#12067=CARTESIAN_POINT ( 'NONE',  ( -92.59262256747321373, 110.5691553257988460, -26.35917033480641436 ) ) ;
#12077=EDGE_CURVE ( 'NONE', #14173, #1119, #4344, .T. ) ;
#12099=DIRECTION ( 'NONE',  ( -2.775557561562890858E-16, -5.724044492823322765E-32, -1.000000000000000000 ) ) ;
#12101=CARTESIAN_POINT ( 'NONE',  ( -107.5926225674731853, 110.5691553257988460, 26.35917033480641436 ) ) ;
#12107=DIRECTION ( 'NONE',  ( -1.000000000000000000, -0.000000000000000000, -0.000000000000000000 ) ) ;
#12122=LINE ( 'NONE', #3500, #11406 ) ;
#12126=ORIENTED_EDGE ( 'NONE', *, *, #14327, .T. ) ;
#12131=EDGE_CURVE ( 'NONE', #12847, #14807, #1446, .T. ) ;
#12152=CARTESIAN_POINT ( 'NONE',  ( -107.5926225674731853, 110.5691553257988460, -26.35917033480641436 ) ) ;
#12158=ORIENTED_EDGE ( 'NONE', *, *, #16810, .F. ) ;
#12161=VERTEX_POINT ( 'NONE', #2859 ) ;
#12172=DIRECTION ( 'NONE',  ( 0.000000000000000000, 1.000000000000000000, 0.000000000000000000 ) ) ;
#12174=ORIENTED_EDGE ( 'NONE', *, *, #11257, .F. ) ;
#12188=CARTESIAN_POINT ( 'NONE',  ( -92.59262256747321373, 110.5691553257988460, 26.35917033480641436 ) ) ;
#12260=AXIS2_PLACEMENT_3D ( 'NONE', #540, #10373, #17474 ) ;
#12278=DIRECTION ( 'NONE',  ( 1.000000000000000000, 0.000000000000000000, -0.000000000000000000 ) ) ;
#12298=ORIENTED_EDGE ( 'NONE', *, *, #10291, .F. ) ;
#12316=CARTESIAN_POINT ( 'NONE',  ( -107.5926225674731995, 60.58224449241411946, -35.00000000000000000 ) ) ;
#12319=ORIENTED_EDGE ( 'NONE', *, *, #2084, .T. ) ;
#12323=VECTOR ( 'NONE', #15931, 1000.000000000000000 ) ;
#12324=ORIENTED_EDGE ( 'NONE', *, *, #10660, .F. ) ;
#12331=AXIS2_PLACEMENT_3D ( 'NONE', #17030, #8253, #2730 ) ;
#12347=AXIS2_PLACEMENT_3D ( 'NONE', #10665, #2045, #3458 ) ;
#12365=CARTESIAN_POINT ( 'NONE',  ( -97.59262256747321373, 106.8071537307723133, -25.00000000000000000 ) ) ;
#12368=CARTESIAN_POINT ( 'NONE',  ( -92.59262256747318531, 0.3328663868096687350, -25.00000000000000000 ) ) ;
#12386=PLANE ( 'NONE',  #10496 ) ;
#12391=ADVANCED_FACE ( 'NONE', ( #8322 ), #3828, .F. ) ;
#12447=VERTEX_POINT ( 'NONE', #10847 ) ;
#12466=EDGE_CURVE ( 'NONE', #10167, #8277, #15709, .T. ) ;
#12475=CARTESIAN_POINT ( 'NONE',  ( -107.5926225674731853, 102.8748711238780373, -20.00000000000000355 ) ) ;
#12538=DIRECTION ( 'NONE',  ( -1.000000000000000000, -0.000000000000000000, -0.000000000000000000 ) ) ;
#12586=( GEOMETRIC_REPRESENTATION_CONTEXT ( 3 ) GLOBAL_UNCERTAINTY_ASSIGNED_CONTEXT ( ( #665 ) ) GLOBAL_UNIT_ASSIGNED_CONTEXT ( ( #5405, #919, #16625 ) ) REPRESENTATION_CONTEXT ( 'NONE', 'WORKASPACE' ) );
#12590=CARTESIAN_POINT ( 'NONE',  ( -107.5926225674732137, 117.8748711238780373, -35.00000000000000000 ) ) ;
#12602=EDGE_CURVE ( 'NONE', #16099, #8042, #3435, .T. ) ;
#12629=VECTOR ( 'NONE', #7832, 1000.000000000000000 ) ;
#12669=CARTESIAN_POINT ( 'NONE',  ( -92.59262256747319952, 61.64996188551983636, 25.00000000000000000 ) ) ;
#12676=EDGE_CURVE ( 'NONE', #6428, #5246, #10276, .T. ) ;
#12694=DIRECTION ( 'NONE',  ( 1.000000000000000000, 2.062304371594500740E-16, -0.000000000000000000 ) ) ;
#12708=AXIS2_PLACEMENT_3D ( 'NONE', #980, #877, #7807 ) ;
#12739=LINE ( 'NONE', #8224, #17706 ) ;
#12746=CARTESIAN_POINT ( 'NONE',  ( -102.5926225674731569, 65.58224449241410525, 20.00000000000000355 ) ) ;
#12771=ORIENTED_EDGE ( 'NONE', *, *, #16401, .T. ) ;
#12788=CARTESIAN_POINT ( 'NONE',  ( -102.5926225674731000, -8.980688996350953114E-14, 0.000000000000000000 ) ) ;
#12811=EDGE_LOOP ( 'NONE', ( #1910, #15856 ) ) ;
#12812=LINE ( 'NONE', #14029, #1005 ) ;
#12823=CARTESIAN_POINT ( 'NONE',  ( -102.5926225674731569, 65.58224449241410525, -20.00000000000000355 ) ) ;
#12847=VERTEX_POINT ( 'NONE', #9172 ) ;
#12868=ORIENTED_EDGE ( 'NONE', *, *, #15449, .T. ) ;
#12871=CARTESIAN_POINT ( 'NONE',  ( -92.59262256747321373, 117.8748711238780373, -35.00000000000000000 ) ) ;
#12874=DIRECTION ( 'NONE',  ( 7.442644330182800165E-16, -1.000000000000000000, 0.000000000000000000 ) ) ;
#12898=ORIENTED_EDGE ( 'NONE', *, *, #4803, .F. ) ;
#12907=ORIENTED_EDGE ( 'NONE', *, *, #10291, .T. ) ;
#12909=CARTESIAN_POINT ( 'NONE',  ( -92.59262256747319952, 57.88796029049330372, 26.35917033480641436 ) ) ;
#12924=DIRECTION ( 'NONE',  ( -1.000000000000000000, -0.000000000000000000, -0.000000000000000000 ) ) ;
#12933=AXIS2_PLACEMENT_3D ( 'NONE', #10160, #8864, #1655 ) ;
#12955=AXIS2_PLACEMENT_3D ( 'NONE', #1062, #3758, #6658 ) ;
#12960=VECTOR ( 'NONE', #8122, 1000.000000000000000 ) ;
#12972=CARTESIAN_POINT ( 'NONE',  ( -92.59262256747321373, 107.8748711238780373, -35.00000000000000000 ) ) ;
#12974=PLANE ( 'NONE',  #9856 ) ;
#12976=EDGE_CURVE ( 'NONE', #17429, #11961, #2221, .T. ) ;
#13004=EDGE_LOOP ( 'NONE', ( #9342, #16790, #13907, #5541 ) ) ;
#13005=DIRECTION ( 'NONE',  ( 0.000000000000000000, 1.000000000000000000, 0.000000000000000000 ) ) ;
#13009=EDGE_LOOP ( 'NONE', ( #4997, #4115, #4875, #7495 ) ) ;
#13053=ADVANCED_FACE ( 'NONE', ( #5290 ), #13882, .F. ) ;
#13062=ORIENTED_EDGE ( 'NONE', *, *, #11909, .T. ) ;
#13080=DIRECTION ( 'NONE',  ( 0.000000000000000000, 1.734723475976811433E-15, 1.000000000000000000 ) ) ;
#13112=EDGE_LOOP ( 'NONE', ( #3807, #5815, #1811, #16492, #4805, #7534 ) ) ;
#13152=ADVANCED_FACE ( 'NONE', ( #5752 ), #4022, .F. ) ;
#13160=VECTOR ( 'NONE', #4192, 1000.000000000000000 ) ;
#13164=EDGE_LOOP ( 'NONE', ( #12898, #4096 ) ) ;
#13185=AXIS2_PLACEMENT_3D ( 'NONE', #2003, #8073, #16493 ) ;
#13197=CARTESIAN_POINT ( 'NONE',  ( -107.5926225674731995, 60.58224449241411946, -35.00000000000000000 ) ) ;
#13224=ORIENTED_EDGE ( 'NONE', *, *, #700, .T. ) ;
#13255=EDGE_CURVE ( 'NONE', #14173, #9962, #1665, .T. ) ;
#13295=EDGE_CURVE ( 'NONE', #5082, #8042, #180, .T. ) ;
#13338=PLANE ( 'NONE',  #5135 ) ;
#13348=ORIENTED_EDGE ( 'NONE', *, *, #1053, .T. ) ;
#13350=FACE_OUTER_BOUND ( 'NONE', #3881, .T. ) ;
#13361=ORIENTED_EDGE ( 'NONE', *, *, #700, .F. ) ;
#13362=CARTESIAN_POINT ( 'NONE',  ( -92.59262256747321373, 106.8071537307723133, 25.00000000000000000 ) ) ;
#13401=DIRECTION ( 'NONE',  ( 0.000000000000000000, 0.000000000000000000, -1.000000000000000000 ) ) ;
#13410=PRODUCT ( '4-Bolt Mounting Plate', '4-Bolt Mounting Plate', '', ( #2363 ) ) ;
#13416=ORIENTED_EDGE ( 'NONE', *, *, #3732, .T. ) ;
#13440=LINE ( 'NONE', #899, #7277 ) ;
#13480=VERTEX_POINT ( 'NONE', #6027 ) ;
#13484=ORIENTED_EDGE ( 'NONE', *, *, #5844, .T. ) ;
#13494=VERTEX_POINT ( 'NONE', #17534 ) ;
#13502=ORIENTED_EDGE ( 'NONE', *, *, #1138, .T. ) ;
#13506=ORIENTED_EDGE ( 'NONE', *, *, #18331, .T. ) ;
#13511=VECTOR ( 'NONE', #7272, 1000.000000000000000 ) ;
#13522=LINE ( 'NONE', #1921, #15580 ) ;
#13527=CIRCLE ( 'NONE', #975, 3.999999999999989786 ) ;
#13536=VECTOR ( 'NONE', #9816, 1000.000000000000000 ) ;
#13567=CYLINDRICAL_SURFACE ( 'NONE', #7815, 3.999999999999989786 ) ;
#13582=EDGE_CURVE ( 'NONE', #12161, #3245, #3158, .T. ) ;
#13603=VERTEX_POINT ( 'NONE', #334 ) ;
#13618=EDGE_CURVE ( 'NONE', #14603, #11466, #4910, .T. ) ;
#13636=DIRECTION ( 'NONE',  ( -1.000000000000000000, -0.000000000000000000, -0.000000000000000000 ) ) ;
#13660=CARTESIAN_POINT ( 'NONE',  ( -107.5926225674731853, 110.5691553257988460, -30.35917033480641081 ) ) ;
#13668=CARTESIAN_POINT ( 'NONE',  ( -107.5926225674731853, 60.58224449241411946, -25.00000000000000000 ) ) ;
#13691=DIRECTION ( 'NONE',  ( 1.000000000000000000, 2.062304371594500740E-16, -0.000000000000000000 ) ) ;
#13701=ORIENTED_EDGE ( 'NONE', *, *, #14067, .T. ) ;
#13717=VECTOR ( 'NONE', #3224, 1000.000000000000000 ) ;
#13731=ORIENTED_EDGE ( 'NONE', *, *, #5154, .F. ) ;
#13739=DIRECTION ( 'NONE',  ( 0.000000000000000000, 0.000000000000000000, -1.000000000000000000 ) ) ;
#13770=CARTESIAN_POINT ( 'NONE',  ( -92.59262256747321373, 117.8748711238780515, -25.00000000000000000 ) ) ;
#13793=LINE ( 'NONE', #5182, #2127 ) ;
#13820=VECTOR ( 'NONE', #2069, 1000.000000000000000 ) ;
#13825=ORIENTED_EDGE ( 'NONE', *, *, #13255, .T. ) ;
#13831=LINE ( 'NONE', #3621, #11957 ) ;
#13833=ORIENTED_EDGE ( 'NONE', *, *, #14235, .T. ) ;
#13857=PLANE ( 'NONE',  #7423 ) ;
#13862=ORIENTED_EDGE ( 'NONE', *, *, #15449, .F. ) ;
#13879=LINE ( 'NONE', #14061, #1573 ) ;
#13882=CONICAL_SURFACE ( 'NONE', #8195, 4.025000000000000355, 0.7853981633974482790 ) ;
#13903=DIRECTION ( 'NONE',  ( 2.062304371594500494E-16, -1.000000000000000000, 0.000000000000000000 ) ) ;
#13906=CARTESIAN_POINT ( 'NONE',  ( -102.5926225674731569, 65.58224449241410525, 20.00000000000000355 ) ) ;
#13907=ORIENTED_EDGE ( 'NONE', *, *, #18104, .F. ) ;
#13939=CARTESIAN_POINT ( 'NONE',  ( -107.5926225674731711, 61.64996188551983636, -25.00000000000000000 ) ) ;
#13951=DIRECTION ( 'NONE',  ( -2.062304371594500494E-16, 1.000000000000000000, -0.000000000000000000 ) ) ;
#13960=DIRECTION ( 'NONE',  ( -1.000000000000000000, -0.000000000000000000, -0.000000000000000000 ) ) ;
#14029=CARTESIAN_POINT ( 'NONE',  ( -107.5926225674731853, 110.5691553257988460, 30.38417033480641294 ) ) ;
#14045=DIRECTION ( 'NONE',  ( 1.000000000000000000, 0.000000000000000000, -0.000000000000000000 ) ) ;
#14052=CARTESIAN_POINT ( 'NONE',  ( -92.59262256747319952, 60.58224449241411946, 35.00000000000000000 ) ) ;
#14061=CARTESIAN_POINT ( 'NONE',  ( -107.5926225674731711, 57.88796029049330372, 22.35917033480642502 ) ) ;
#14067=EDGE_CURVE ( 'NONE', #14807, #14603, #7929, .T. ) ;
#14077=STYLED_ITEM('',(#18566),#6235);
#14081=VECTOR ( 'NONE', #7515, 1000.000000000000000 ) ;
#14085=PLANE ( 'NONE',  #1866 ) ;
#14088=DIRECTION ( 'NONE',  ( -1.000000000000000000, 0.000000000000000000, -0.000000000000000000 ) ) ;
#14091=EDGE_CURVE ( 'NONE', #7683, #4700, #6743, .T. ) ;
#14123=VERTEX_POINT ( 'NONE', #4040 ) ;
#14171=ADVANCED_BREP_SHAPE_REPRESENTATION ( '', ( #6235, #16217 ), #3695 ) ;
#14173=VERTEX_POINT ( 'NONE', #11253 ) ;
#14235=EDGE_CURVE ( 'NONE', #13480, #16207, #11690, .T. ) ;
#14239=ADVANCED_FACE ( 'NONE', ( #14580 ), #16156, .T. ) ;
#14246=ORIENTED_EDGE ( 'NONE', *, *, #4795, .T. ) ;
#14248=LINE ( 'NONE', #9935, #2805 ) ;
#14256=PLANE ( 'NONE',  #3576 ) ;
#14275=VERTEX_POINT ( 'NONE', #3447 ) ;
#14280=VERTEX_POINT ( 'NONE', #13362 ) ;
#14289=CARTESIAN_POINT ( 'NONE',  ( -97.59262256747318531, 57.88796029049330372, 22.35917033480642502 ) ) ;
#14296=LINE ( 'NONE', #6006, #14081 ) ;
#14301=ADVANCED_FACE ( 'NONE', ( #14501 ), #10170, .F. ) ;
#14327=EDGE_CURVE ( 'NONE', #3086, #2130, #13831, .T. ) ;
#14343=VECTOR ( 'NONE', #3467, 1000.000000000000000 ) ;
#14349=ORIENTED_EDGE ( 'NONE', *, *, #12077, .T. ) ;
#14357=ORIENTED_EDGE ( 'NONE', *, *, #9255, .T. ) ;
#14419=DIRECTION ( 'NONE',  ( -7.442644330182800165E-16, 1.000000000000000000, 0.000000000000000000 ) ) ;
#14423=EDGE_CURVE ( 'NONE', #857, #15190, #8681, .T. ) ;
#14425=ORIENTED_EDGE ( 'NONE', *, *, #18069, .T. ) ;
#14431=CONICAL_SURFACE ( 'NONE', #15620, 4.025000000000000355, 0.7853981633974482790 ) ;
#14473=FACE_OUTER_BOUND ( 'NONE', #6968, .T. ) ;
#14477=AXIS2_PLACEMENT_3D ( 'NONE', #1457, #7160, #5113 ) ;
#14479=CIRCLE ( 'NONE', #3400, 4.025000000000000355 ) ;
#14481=CIRCLE ( 'NONE', #15967, 4.025000000000000355 ) ;
#14488=DIRECTION ( 'NONE',  ( 1.000000000000000000, 2.062304371594500494E-16, 0.000000000000000000 ) ) ;
#14501=FACE_OUTER_BOUND ( 'NONE', #7625, .T. ) ;
#14519=FACE_OUTER_BOUND ( 'NONE', #13004, .T. ) ;
#14529=CARTESIAN_POINT ( 'NONE',  ( -107.5676225674731938, 110.5691553257988460, 26.35917033480641436 ) ) ;
#14530=ORIENTED_EDGE ( 'NONE', *, *, #2053, .T. ) ;
#14547=LINE ( 'NONE', #4793, #9090 ) ;
#14580=FACE_OUTER_BOUND ( 'NONE', #10107, .T. ) ;
#14595=PLANE ( 'NONE',  #11115 ) ;
#14603=VERTEX_POINT ( 'NONE', #14731 ) ;
#14607=CARTESIAN_POINT ( 'NONE',  ( -107.5676225674731654, 57.88796029049330372, -22.35917033480641791 ) ) ;
#14721=CARTESIAN_POINT ( 'NONE',  ( -107.5926225674731853, 110.5691553257988460, 30.38417033480641294 ) ) ;
#14731=CARTESIAN_POINT ( 'NONE',  ( -107.5926225674731853, 50.58224449241411236, -25.00000000000000000 ) ) ;
#14740=ORIENTED_EDGE ( 'NONE', *, *, #7904, .T. ) ;
#14806=FACE_OUTER_BOUND ( 'NONE', #193, .T. ) ;
#14807=VERTEX_POINT ( 'NONE', #12316 ) ;
#14815=FACE_OUTER_BOUND ( 'NONE', #8451, .T. ) ;
#14831=ADVANCED_FACE ( 'NONE', ( #3506 ), #14909, .F. ) ;
#14864=DIRECTION ( 'NONE',  ( -1.000000000000000000, -0.000000000000000000, -0.000000000000000000 ) ) ;
#14883=CARTESIAN_POINT ( 'NONE',  ( -107.5676225674731654, 57.88796029049330372, -26.35917033480641436 ) ) ;
#14904=CIRCLE ( 'NONE', #17305, 3.999999999999989786 ) ;
#14909=CYLINDRICAL_SURFACE ( 'NONE', #1809, 3.999999999999989786 ) ;
#14915=VERTEX_POINT ( 'NONE', #8296 ) ;
#14932=AXIS2_PLACEMENT_3D ( 'NONE', #3009, #7395, #6240 ) ;
#14987=FACE_OUTER_BOUND ( 'NONE', #5688, .T. ) ;
#15011=ORIENTED_EDGE ( 'NONE', *, *, #47, .F. ) ;
#15060=FACE_OUTER_BOUND ( 'NONE', #13009, .T. ) ;
#15082=VECTOR ( 'NONE', #8026, 1000.000000000000000 ) ;
#15085=DIRECTION ( 'NONE',  ( 0.000000000000000000, 0.000000000000000000, 1.000000000000000000 ) ) ;
#15104=DIRECTION ( 'NONE',  ( -2.062304371594500494E-16, 1.000000000000000000, -0.000000000000000000 ) ) ;
#15116=DIRECTION ( 'NONE',  ( 0.000000000000000000, 0.000000000000000000, 1.000000000000000000 ) ) ;
#15131=DIRECTION ( 'NONE',  ( 1.000000000000000000, 2.062304371594500494E-16, -2.775557561562890858E-16 ) ) ;
#15133=ORIENTED_EDGE ( 'NONE', *, *, #9981, .T. ) ;
#15157=PLANE ( 'NONE',  #3355 ) ;
#15165=ORIENTED_EDGE ( 'NONE', *, *, #2184, .T. ) ;
#15189=CARTESIAN_POINT ( 'NONE',  ( -102.5926225674731853, 102.8748711238780373, -20.00000000000000355 ) ) ;
#15190=VERTEX_POINT ( 'NONE', #16650 ) ;
#15199=CARTESIAN_POINT ( 'NONE',  ( -107.5926225674731711, 57.88796029049330372, -26.35917033480641436 ) ) ;
#15206=EDGE_CURVE ( 'NONE', #3086, #6428, #2690, .T. ) ;
#15212=ADVANCED_FACE ( 'NONE', ( #9464 ), #15259, .F. ) ;
#15234=CARTESIAN_POINT ( 'NONE',  ( -107.5926225674731711, 57.88796029049330372, -30.35917033480640370 ) ) ;
#15245=VERTEX_POINT ( 'NONE', #2260 ) ;
#15259=PLANE ( 'NONE',  #16108 ) ;
#15263=DIRECTION ( 'NONE',  ( 0.000000000000000000, 0.000000000000000000, 1.000000000000000000 ) ) ;
#15270=AXIS2_PLACEMENT_3D ( 'NONE', #16882, #12694, #11285 ) ;
#15281=VECTOR ( 'NONE', #13401, 1000.000000000000000 ) ;
#15330=CARTESIAN_POINT ( 'NONE',  ( -97.59262256747321373, 117.8748711238780515, -25.00000000000000000 ) ) ;
#15333=VERTEX_POINT ( 'NONE', #12669 ) ;
#15351=CARTESIAN_POINT ( 'NONE',  ( -92.59262256747318531, 0.3328663868096687350, 25.00000000000000000 ) ) ;
#15357=EDGE_LOOP ( 'NONE', ( #11069, #3108, #2545, #10897, #10633, #2989, #11738, #5982, #14349, #13416, #17562, #7729, #11783, #13731, #11762, #4728 ) ) ;
#15358=AXIS2_PLACEMENT_3D ( 'NONE', #6801, #11016, #7825 ) ;
#15369=CYLINDRICAL_SURFACE ( 'NONE', #7510, 9.999999999999994671 ) ;
#15388=SHAPE_DEFINITION_REPRESENTATION ( #11040, #16862 ) ;
#15444=ORIENTED_EDGE ( 'NONE', *, *, #18104, .T. ) ;
#15449=EDGE_CURVE ( 'NONE', #6428, #3086, #4756, .T. ) ;
#15459=DIRECTION ( 'NONE',  ( 0.000000000000000000, 0.000000000000000000, 1.000000000000000000 ) ) ;
#15464=CARTESIAN_POINT ( 'NONE',  ( -97.59262256747319952, 50.58224449241411236, -25.00000000000000000 ) ) ;
#15465=ADVANCED_FACE ( 'NONE', ( #11610 ), #3356, .T. ) ;
#15479=DIRECTION ( 'NONE',  ( 2.062304371594500494E-16, -1.000000000000000000, 0.000000000000000000 ) ) ;
#15500=DIRECTION ( 'NONE',  ( -0.000000000000000000, 0.000000000000000000, -1.000000000000000000 ) ) ;
#15512=ORIENTED_EDGE ( 'NONE', *, *, #17197, .F. ) ;
#15538=CARTESIAN_POINT ( 'NONE',  ( -107.5926225674731853, 110.5691553257988460, 26.35917033480641436 ) ) ;
#15562=ORIENTED_EDGE ( 'NONE', *, *, #17734, .F. ) ;
#15575=EDGE_CURVE ( 'NONE', #16660, #6428, #4851, .T. ) ;
#15580=VECTOR ( 'NONE', #10518, 1000.000000000000000 ) ;
#15603=ORIENTED_EDGE ( 'NONE', *, *, #7344, .T. ) ;
#15620=AXIS2_PLACEMENT_3D ( 'NONE', #15538, #13960, #2636 ) ;
#15623=DIRECTION ( 'NONE',  ( -0.7071067811864494290, 8.659560562356134638E-17, -0.7071067811866454944 ) ) ;
#15632=DIRECTION ( 'NONE',  ( 0.000000000000000000, 0.000000000000000000, 1.000000000000000000 ) ) ;
#15651=VECTOR ( 'NONE', #13739, 1000.000000000000000 ) ;
#15656=DIRECTION ( 'NONE',  ( 0.000000000000000000, 0.000000000000000000, 1.000000000000000000 ) ) ;
#15658=ORIENTED_EDGE ( 'NONE', *, *, #7596, .T. ) ;
#15663=ORIENTED_EDGE ( 'NONE', *, *, #4795, .F. ) ;
#15686=ORIENTED_EDGE ( 'NONE', *, *, #18437, .T. ) ;
#15697=ORIENTED_EDGE ( 'NONE', *, *, #2053, .F. ) ;
#15706=CARTESIAN_POINT ( 'NONE',  ( -92.59262256747321373, 110.5691553257988460, 30.35917033480641081 ) ) ;
#15709=CIRCLE ( 'NONE', #3737, 9.999999999999994671 ) ;
#15719=DIRECTION ( 'NONE',  ( -2.062304371594500494E-16, 1.000000000000000000, -0.000000000000000000 ) ) ;
#15730=DIRECTION ( 'NONE',  ( 0.000000000000000000, 1.000000000000000000, 0.000000000000000000 ) ) ;
#15738=DIRECTION ( 'NONE',  ( 0.000000000000000000, 0.000000000000000000, 1.000000000000000000 ) ) ;
#15752=CARTESIAN_POINT ( 'NONE',  ( -107.5926225674732137, 117.8748711238780373, -25.00000000000000000 ) ) ;
#15770=LINE ( 'NONE', #4437, #6357 ) ;
#15839=LINE ( 'NONE', #9870, #4792 ) ;
#15850=EDGE_CURVE ( 'NONE', #11731, #9165, #10366, .T. ) ;
#15853=DIRECTION ( 'NONE',  ( -2.062304371594500494E-16, 1.000000000000000000, -0.000000000000000000 ) ) ;
#15856=ORIENTED_EDGE ( 'NONE', *, *, #17965, .F. ) ;
#15865=CARTESIAN_POINT ( 'NONE',  ( -97.59262256747318531, 57.88796029049330372, 26.35917033480641436 ) ) ;
#15882=AXIS2_PLACEMENT_3D ( 'NONE', #17162, #8648, #1632 ) ;
#15893=VECTOR ( 'NONE', #17531, 1000.000000000000000 ) ;
#15907=CIRCLE ( 'NONE', #1570, 3.999999999999989786 ) ;
#15926=VECTOR ( 'NONE', #14419, 1000.000000000000000 ) ;
#15931=DIRECTION ( 'NONE',  ( 1.000000000000000000, 0.000000000000000000, 0.000000000000000000 ) ) ;
#15939=DIRECTION ( 'NONE',  ( 1.000000000000000000, 2.062304371594500740E-16, 0.000000000000000000 ) ) ;
#15961=CIRCLE ( 'NONE', #1926, 9.999999999999994671 ) ;
#15966=ORIENTED_EDGE ( 'NONE', *, *, #17173, .F. ) ;
#15967=AXIS2_PLACEMENT_3D ( 'NONE', #3937, #9756, #2553 ) ;
#15980=DIRECTION ( 'NONE',  ( -0.7071067811864494290, 8.659560562356134638E-17, -0.7071067811866454944 ) ) ;
#16013=ADVANCED_FACE ( 'NONE', ( #12048, #16520, #1944, #904, #3718, #6221 ), #2216, .F. ) ;
#16031=ORIENTED_EDGE ( 'NONE', *, *, #16836, .F. ) ;
#16065=ORIENTED_EDGE ( 'NONE', *, *, #4139, .F. ) ;
#16086=ORIENTED_EDGE ( 'NONE', *, *, #2084, .F. ) ;
#16099=VERTEX_POINT ( 'NONE', #10548 ) ;
#16108=AXIS2_PLACEMENT_3D ( 'NONE', #16745, #3845, #12278 ) ;
#16117=CARTESIAN_POINT ( 'NONE',  ( -107.5676225674731938, 110.5691553257988460, 22.35917033480641081 ) ) ;
#16124=LINE ( 'NONE', #4907, #15893 ) ;
#16125=CARTESIAN_POINT ( 'NONE',  ( -92.59262256747318531, 50.58224449241411236, -25.00000000000000000 ) ) ;
#16156=PLANE ( 'NONE',  #17621 ) ;
#16199=ADVANCED_FACE ( 'NONE', ( #11216 ), #16905, .F. ) ;
#16203=AXIS2_PLACEMENT_3D ( 'NONE', #12067, #9348, #9078 ) ;
#16207=VERTEX_POINT ( 'NONE', #1009 ) ;
#16217=AXIS2_PLACEMENT_3D ( 'NONE', #5781, #6037, #8961 ) ;
#16276=DIRECTION ( 'NONE',  ( 0.000000000000000000, 0.000000000000000000, 1.000000000000000000 ) ) ;
#16293=CARTESIAN_POINT ( 'NONE',  ( -107.5926225674731853, 50.58224449241411236, 35.00000000000000000 ) ) ;
#16306=DIRECTION ( 'NONE',  ( 1.000000000000000000, 2.062304371594500494E-16, -2.775557561562890858E-16 ) ) ;
#16308=CYLINDRICAL_SURFACE ( 'NONE', #13185, 3.999999999999996447 ) ;
#16350=LINE ( 'NONE', #4847, #11792 ) ;
#16367=EDGE_CURVE ( 'NONE', #12161, #9136, #12122, .T. ) ;
#16378=CARTESIAN_POINT ( 'NONE',  ( -107.5926225674731711, 57.88796029049330372, 26.35917033480641436 ) ) ;
#16379=CARTESIAN_POINT ( 'NONE',  ( -97.59262256747319952, 50.58224449241411236, -25.00000000000000000 ) ) ;
#16397=ORIENTED_EDGE ( 'NONE', *, *, #15575, .F. ) ;
#16401=EDGE_CURVE ( 'NONE', #4700, #2247, #13522, .T. ) ;
#16405=CARTESIAN_POINT ( 'NONE',  ( -107.5926225674731711, 57.88796029049330372, -26.35917033480641436 ) ) ;
#16412=VECTOR ( 'NONE', #3168, 1000.000000000000000 ) ;
#16431=VERTEX_POINT ( 'NONE', #17718 ) ;
#16441=LINE ( 'NONE', #3632, #1603 ) ;
#16462=EDGE_CURVE ( 'NONE', #11084, #2797, #17070, .T. ) ;
#16490=DIRECTION ( 'NONE',  ( 0.000000000000000000, 1.000000000000000000, 0.000000000000000000 ) ) ;
#16492=ORIENTED_EDGE ( 'NONE', *, *, #5514, .F. ) ;
#16493=DIRECTION ( 'NONE',  ( 0.000000000000000000, 0.000000000000000000, 1.000000000000000000 ) ) ;
#16513=CIRCLE ( 'NONE', #18338, 4.025000000000000355 ) ;
#16520=FACE_BOUND ( 'NONE', #9293, .T. ) ;
#16536=ORIENTED_EDGE ( 'NONE', *, *, #11257, .T. ) ;
#16553=EDGE_LOOP ( 'NONE', ( #971, #15444, #15165, #542 ) ) ;
#16566=ORIENTED_EDGE ( 'NONE', *, *, #8223, .T. ) ;
#16608=CARTESIAN_POINT ( 'NONE',  ( -107.5676225674731938, 110.5691553257988460, -26.35917033480641436 ) ) ;
#16625=( NAMED_UNIT ( * ) SI_UNIT ( $, .STERADIAN. ) SOLID_ANGLE_UNIT ( ) );
#16631=FACE_OUTER_BOUND ( 'NONE', #2818, .T. ) ;
#16633=DIRECTION ( 'NONE',  ( -1.000000000000000000, -0.000000000000000000, -0.000000000000000000 ) ) ;
#16650=CARTESIAN_POINT ( 'NONE',  ( -97.59262256747319952, 54.12595869546677818, -25.00000000000000000 ) ) ;
#16660=VERTEX_POINT ( 'NONE', #8284 ) ;
#16674=ORIENTED_EDGE ( 'NONE', *, *, #10618, .T. ) ;
#16678=ADVANCED_FACE ( 'NONE', ( #6971 ), #6872, .T. ) ;
#16686=VECTOR ( 'NONE', #13636, 1000.000000000000000 ) ;
#16722=DIRECTION ( 'NONE',  ( -2.062304371594500247E-16, 1.000000000000000000, 0.000000000000000000 ) ) ;
#16737=ORIENTED_EDGE ( 'NONE', *, *, #1920, .T. ) ;
#16745=CARTESIAN_POINT ( 'NONE',  ( -107.5926225674732137, 117.8748711238780373, -35.00000000000000000 ) ) ;
#16748=ORIENTED_EDGE ( 'NONE', *, *, #17582, .F. ) ;
#16750=FACE_OUTER_BOUND ( 'NONE', #8305, .T. ) ;
#16756=DIRECTION ( 'NONE',  ( -0.7071067811865474617, 8.659560562354932858E-17, -0.7071067811865474617 ) ) ;
#16769=CONICAL_SURFACE ( 'NONE', #5427, 4.025000000000000355, 0.7853981633974482790 ) ;
#16772=DIRECTION ( 'NONE',  ( -2.062304371594500494E-16, 1.000000000000000000, -0.000000000000000000 ) ) ;
#16779=PLANE ( 'NONE',  #3874 ) ;
#16790=ORIENTED_EDGE ( 'NONE', *, *, #9703, .F. ) ;
#16810=EDGE_CURVE ( 'NONE', #16660, #13494, #9314, .T. ) ;
#16825=EDGE_CURVE ( 'NONE', #5132, #10461, #5061, .T. ) ;
#16836=EDGE_CURVE ( 'NONE', #14123, #14915, #3568, .T. ) ;
#16848=AXIS2_PLACEMENT_3D ( 'NONE', #11262, #1239, #16950 ) ;
#16862=SHAPE_REPRESENTATION ( '4-Bolt Mounting Plate', ( #16217 ), #3695 ) ;
#16879=CARTESIAN_POINT ( 'NONE',  ( -97.59262256747318531, 0.3328663868096687350, -25.00000000000000000 ) ) ;
#16880=ORIENTED_EDGE ( 'NONE', *, *, #1053, .F. ) ;
#16882=CARTESIAN_POINT ( 'NONE',  ( -107.5926225674732137, 107.8748711238780373, -25.00000000000000000 ) ) ;
#16885=FACE_OUTER_BOUND ( 'NONE', #7789, .T. ) ;
#16905=PLANE ( 'NONE',  #5081 ) ;
#16918=ORIENTED_EDGE ( 'NONE', *, *, #993, .F. ) ;
#16922=ADVANCED_FACE ( 'NONE', ( #7693 ), #16769, .F. ) ;
#16924=DIRECTION ( 'NONE',  ( 0.000000000000000000, 0.000000000000000000, 1.000000000000000000 ) ) ;
#16926=EDGE_CURVE ( 'NONE', #12020, #9165, #404, .T. ) ;
#16927=EDGE_LOOP ( 'NONE', ( #4620, #18100, #17633, #5694 ) ) ;
#16943=ORIENTED_EDGE ( 'NONE', *, *, #1140, .F. ) ;
#16950=DIRECTION ( 'NONE',  ( 0.000000000000000000, 0.000000000000000000, 1.000000000000000000 ) ) ;
#16962=ADVANCED_FACE ( 'NONE', ( #5161 ), #12386, .F. ) ;
#16970=CARTESIAN_POINT ( 'NONE',  ( -107.5926225674731853, 114.3311569208253786, 25.00000000000000000 ) ) ;
#17003=CARTESIAN_POINT ( 'NONE',  ( -107.5926225674731853, 50.58224449241411236, 25.00000000000000000 ) ) ;
#17009=CARTESIAN_POINT ( 'NONE',  ( -107.5926225674731853, 106.8071537307723133, 25.00000000000000000 ) ) ;
#17030=CARTESIAN_POINT ( 'NONE',  ( -107.5926225674731853, 107.8748711238780373, 25.00000000000000000 ) ) ;
#17035=CARTESIAN_POINT ( 'NONE',  ( -107.5676225674731654, 57.88796029049330372, -26.35917033480641436 ) ) ;
#17062=ADVANCED_FACE ( 'NONE', ( #16750 ), #15369, .T. ) ;
#17070=CIRCLE ( 'NONE', #322, 3.999999999999996447 ) ;
#17076=ORIENTED_EDGE ( 'NONE', *, *, #13582, .T. ) ;
#17103=VECTOR ( 'NONE', #11551, 1000.000000000000000 ) ;
#17122=AXIS2_PLACEMENT_3D ( 'NONE', #16608, #4819, #15116 ) ;
#17162=CARTESIAN_POINT ( 'NONE',  ( -92.59262256747319952, 57.88796029049330372, -26.35917033480641436 ) ) ;
#17173=EDGE_CURVE ( 'NONE', #18159, #9136, #4937, .T. ) ;
#17197=EDGE_CURVE ( 'NONE', #3821, #14173, #10647, .T. ) ;
#17209=DIRECTION ( 'NONE',  ( -1.000000000000000000, -2.062304371594500247E-16, -0.000000000000000000 ) ) ;
#17217=ORIENTED_EDGE ( 'NONE', *, *, #18461, .T. ) ;
#17241=DIRECTION ( 'NONE',  ( 0.000000000000000000, 1.000000000000000000, 0.000000000000000000 ) ) ;
#17245=ORIENTED_EDGE ( 'NONE', *, *, #17965, .T. ) ;
#17274=EDGE_LOOP ( 'NONE', ( #17668, #16918, #3693, #2823 ) ) ;
#17279=( NAMED_UNIT ( * ) SI_UNIT ( $, .STERADIAN. ) SOLID_ANGLE_UNIT ( ) );
#17305=AXIS2_PLACEMENT_3D ( 'NONE', #3212, #17798, #9017 ) ;
#17313=ORIENTED_EDGE ( 'NONE', *, *, #12602, .T. ) ;
#17316=VERTEX_POINT ( 'NONE', #15706 ) ;
#17320=DIRECTION ( 'NONE',  ( 0.000000000000000000, 0.000000000000000000, 1.000000000000000000 ) ) ;
#17326=CARTESIAN_POINT ( 'NONE',  ( -107.5926225674732137, 107.8748711238780373, -35.00000000000000000 ) ) ;
#17330=FACE_OUTER_BOUND ( 'NONE', #16553, .T. ) ;
#17339=ORIENTED_EDGE ( 'NONE', *, *, #993, .T. ) ;
#17381=EDGE_CURVE ( 'NONE', #8404, #3000, #9038, .T. ) ;
#17429=VERTEX_POINT ( 'NONE', #16125 ) ;
#17436=CIRCLE ( 'NONE', #15358, 3.999999999999989786 ) ;
#17440=DIRECTION ( 'NONE',  ( -1.000000000000000000, -0.000000000000000000, -0.000000000000000000 ) ) ;
#17443=DIRECTION ( 'NONE',  ( 1.000000000000000000, 2.062304371594500494E-16, -2.775557561562890858E-16 ) ) ;
#17445=EDGE_CURVE ( 'NONE', #9165, #14123, #3054, .T. ) ;
#17446=ORIENTED_EDGE ( 'NONE', *, *, #9244, .T. ) ;
#17474=DIRECTION ( 'NONE',  ( 0.000000000000000000, 0.000000000000000000, 1.000000000000000000 ) ) ;
#17492=ADVANCED_FACE ( 'NONE', ( #14473 ), #1561, .F. ) ;
#17495=EDGE_CURVE ( 'NONE', #10265, #11747, #10509, .T. ) ;
#17504=ORIENTED_EDGE ( 'NONE', *, *, #14067, .F. ) ;
#17511=DIRECTION ( 'NONE',  ( 0.000000000000000000, 0.000000000000000000, 1.000000000000000000 ) ) ;
#17531=DIRECTION ( 'NONE',  ( 1.000000000000000000, 0.000000000000000000, 0.000000000000000000 ) ) ;
#17534=CARTESIAN_POINT ( 'NONE',  ( -92.59262256747319952, 61.64996188551983636, -25.00000000000000000 ) ) ;
#17562=ORIENTED_EDGE ( 'NONE', *, *, #1138, .F. ) ;
#17571=DIRECTION ( 'NONE',  ( 2.775557561562890858E-16, 0.000000000000000000, 1.000000000000000000 ) ) ;
#17582=EDGE_CURVE ( 'NONE', #11731, #3038, #6398, .T. ) ;
#17585=CYLINDRICAL_SURFACE ( 'NONE', #8515, 3.999999999999996447 ) ;
#17590=ORIENTED_EDGE ( 'NONE', *, *, #14327, .F. ) ;
#17621=AXIS2_PLACEMENT_3D ( 'NONE', #1956, #1763, #11866 ) ;
#17633=ORIENTED_EDGE ( 'NONE', *, *, #6273, .T. ) ;
#17635=DIRECTION ( 'NONE',  ( -1.000000000000000000, -2.062304371594500740E-16, -0.000000000000000000 ) ) ;
#17668=ORIENTED_EDGE ( 'NONE', *, *, #1081, .F. ) ;
#17700=CIRCLE ( 'NONE', #12955, 4.025000000000000355 ) ;
#17706=VECTOR ( 'NONE', #15719, 1000.000000000000000 ) ;
#17711=CARTESIAN_POINT ( 'NONE',  ( -97.59262256747321373, 110.5691553257988460, -26.35917033480641436 ) ) ;
#17715=DIRECTION ( 'NONE',  ( -0.7071067811864494290, 0.000000000000000000, 0.7071067811866454944 ) ) ;
#17718=CARTESIAN_POINT ( 'NONE',  ( -97.59262256747319952, 110.5691553257988460, 22.35917033480641791 ) ) ;
#17734=EDGE_CURVE ( 'NONE', #18456, #14915, #2480, .T. ) ;
#17745=ORIENTED_EDGE ( 'NONE', *, *, #11565, .F. ) ;
#17773=EDGE_LOOP ( 'NONE', ( #8964, #545, #1078, #16737 ) ) ;
#17783=CARTESIAN_POINT ( 'NONE',  ( -92.59262256747318531, 0.3328663868096687350, 25.00000000000000000 ) ) ;
#17796=FACE_OUTER_BOUND ( 'NONE', #3706, .T. ) ;
#17798=DIRECTION ( 'NONE',  ( 1.000000000000000000, 2.062304371594500494E-16, 0.000000000000000000 ) ) ;
#17815=ADVANCED_FACE ( 'NONE', ( #5287 ), #9461, .F. ) ;
#17818=ORIENTED_EDGE ( 'NONE', *, *, #8912, .F. ) ;
#17822=EDGE_CURVE ( 'NONE', #10461, #17429, #5250, .T. ) ;
#17828=DIRECTION ( 'NONE',  ( -2.062304371594500494E-16, 1.000000000000000000, -0.000000000000000000 ) ) ;
#17839=DIRECTION ( 'NONE',  ( -1.000000000000000000, -0.000000000000000000, -0.000000000000000000 ) ) ;
#17863=ORIENTED_EDGE ( 'NONE', *, *, #18144, .F. ) ;
#17904=DIRECTION ( 'NONE',  ( -1.000000000000000000, -0.000000000000000000, -0.000000000000000000 ) ) ;
#17949=ORIENTED_EDGE ( 'NONE', *, *, #9255, .F. ) ;
#17953=ADVANCED_FACE ( 'NONE', ( #4051 ), #14431, .F. ) ;
#17958=EDGE_CURVE ( 'NONE', #9136, #8404, #9343, .T. ) ;
#17965=EDGE_CURVE ( 'NONE', #13603, #11807, #6035, .T. ) ;
#17975=CARTESIAN_POINT ( 'NONE',  ( -92.59262256747318531, 0.3328663868096687350, 25.00000000000000000 ) ) ;
#18040=LINE ( 'NONE', #9345, #15651 ) ;
#18051=CARTESIAN_POINT ( 'NONE',  ( -102.5926225674731853, 102.8748711238780373, 20.00000000000000355 ) ) ;
#18069=EDGE_CURVE ( 'NONE', #3821, #8277, #14248, .T. ) ;
#18093=ORIENTED_EDGE ( 'NONE', *, *, #9981, .F. ) ;
#18097=CARTESIAN_POINT ( 'NONE',  ( -92.59262256747319952, 60.58224449241411946, 25.00000000000000000 ) ) ;
#18100=ORIENTED_EDGE ( 'NONE', *, *, #16825, .F. ) ;
#18104=EDGE_CURVE ( 'NONE', #18456, #18220, #3262, .T. ) ;
#18144=EDGE_CURVE ( 'NONE', #11961, #14807, #3094, .T. ) ;
#18158=EDGE_LOOP ( 'NONE', ( #17504, #17863, #2914, #5978, #5944 ) ) ;
#18159=VERTEX_POINT ( 'NONE', #6148 ) ;
#18166=DIRECTION ( 'NONE',  ( -1.000000000000000000, -0.000000000000000000, -0.000000000000000000 ) ) ;
#18220=VERTEX_POINT ( 'NONE', #10202 ) ;
#18263=CARTESIAN_POINT ( 'NONE',  ( -107.5926225674731853, 110.5691553257988460, -26.35917033480641436 ) ) ;
#18295=ORIENTED_EDGE ( 'NONE', *, *, #16401, .F. ) ;
#18301=EDGE_CURVE ( 'NONE', #2247, #2087, #11458, .T. ) ;
#18321=DIRECTION ( 'NONE',  ( 0.000000000000000000, 3.469446951953617344E-15, 1.000000000000000000 ) ) ;
#18331=EDGE_CURVE ( 'NONE', #11747, #7063, #6052, .T. ) ;
#18338=AXIS2_PLACEMENT_3D ( 'NONE', #6949, #18373, #15656 ) ;
#18341=ORIENTED_EDGE ( 'NONE', *, *, #6649, .T. ) ;
#18349=DIRECTION ( 'NONE',  ( 0.000000000000000000, 1.000000000000000000, 0.000000000000000000 ) ) ;
#18369=ORIENTED_EDGE ( 'NONE', *, *, #8912, .T. ) ;
#18373=DIRECTION ( 'NONE',  ( -1.000000000000000000, -0.000000000000000000, -0.000000000000000000 ) ) ;
#18391=VECTOR ( 'NONE', #2519, 1000.000000000000000 ) ;
#18396=DIRECTION ( 'NONE',  ( -2.062304371594500494E-16, 1.000000000000000000, 0.000000000000000000 ) ) ;
#18402=AXIS2_PLACEMENT_3D ( 'NONE', #13668, #2150, #12172 ) ;
#18437=EDGE_CURVE ( 'NONE', #13494, #7683, #4019, .T. ) ;
#18448=ADVANCED_FACE ( 'NONE', ( #16631 ), #3823, .F. ) ;
#18451=ORIENTED_EDGE ( 'NONE', *, *, #2375, .F. ) ;
#18456=VERTEX_POINT ( 'NONE', #12746 ) ;
#18457=PRODUCT_DEFINITION_CONTEXT ( 'detailed design', #8738, 'design' ) ;
#18461=EDGE_CURVE ( 'NONE', #11084, #2867, #11320, .T. ) ;
#18484=FACE_OUTER_BOUND ( 'NONE', #3887, .T. ) ;
#18488=DIRECTION ( 'NONE',  ( -1.000000000000000000, -0.000000000000000000, -0.000000000000000000 ) ) ;
#18492=ORIENTED_EDGE ( 'NONE', *, *, #5514, .T. ) ;
#18560=COLOUR_RGB('Black',0.12,0.14,0.17);
#18561=FILL_AREA_STYLE_COLOUR('',#18560);
#18562=FILL_AREA_STYLE('',(#18561));
#18563=SURFACE_STYLE_FILL_AREA(#18562);
#18564=SURFACE_SIDE_STYLE('',(#18563));
#18565=SURFACE_STYLE_USAGE(.BOTH.,#18564);
#18566=PRESENTATION_STYLE_ASSIGNMENT((#18565));
ENDSEC;
END-ISO-10303-21;
